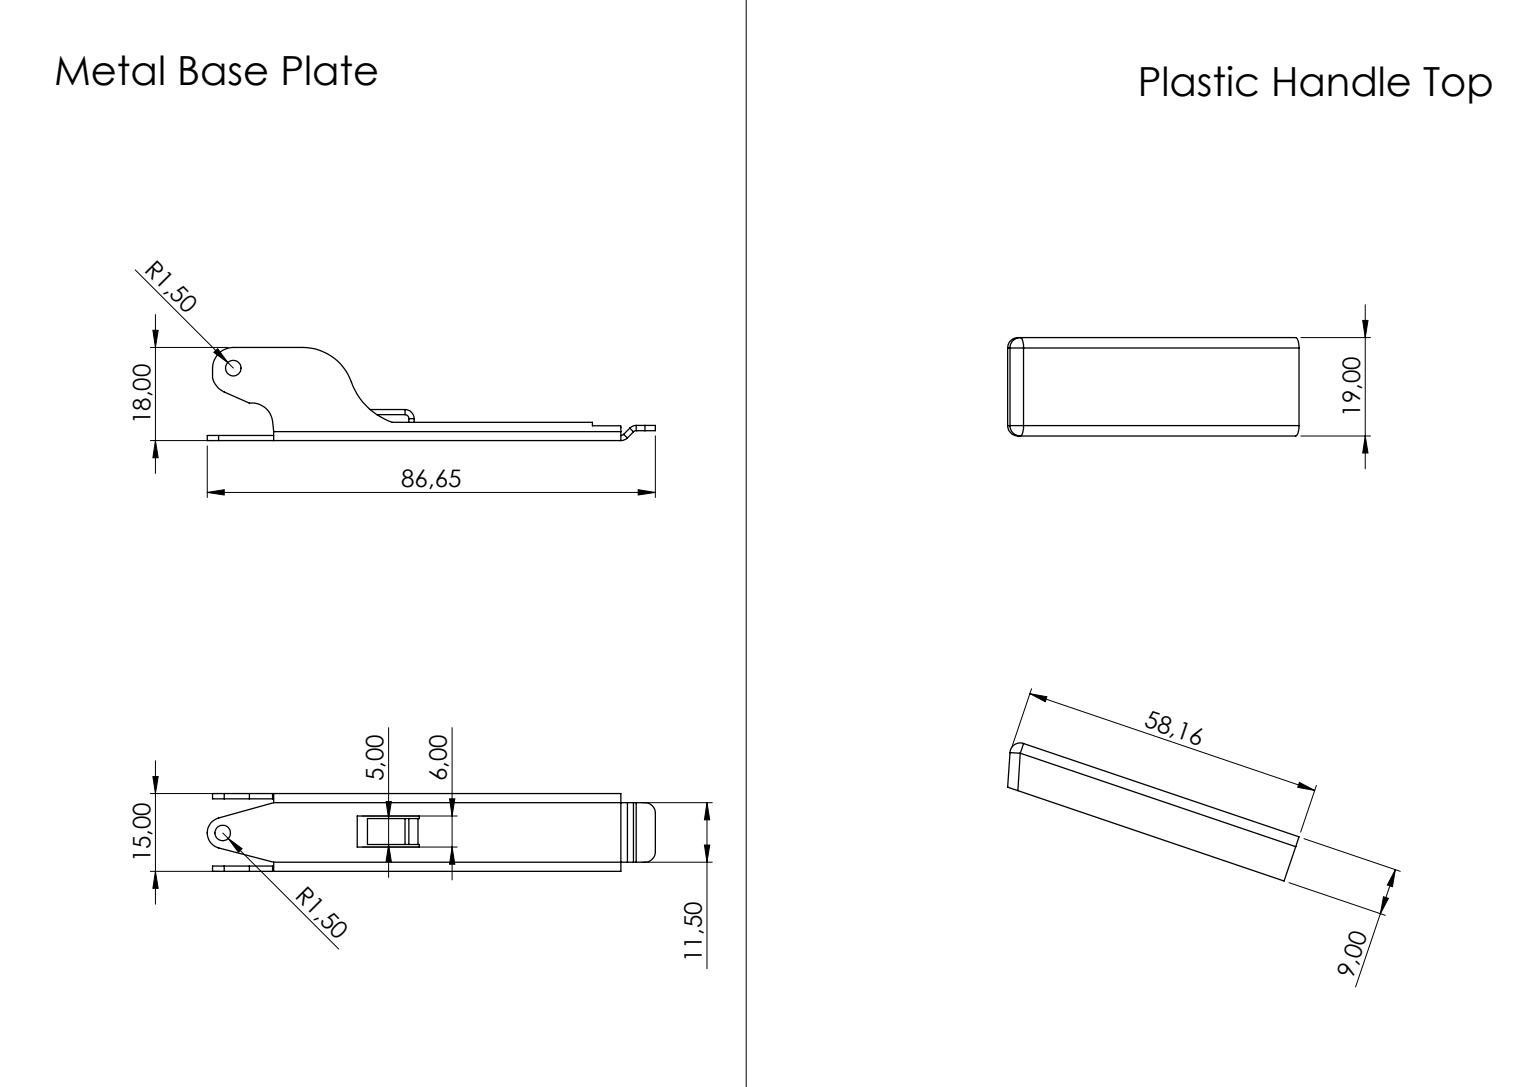
ISO-10303-21;
HEADER;
FILE_DESCRIPTION (('STEP AP214'),
    '1' );
FILE_NAME ('Metal Base Plate.step',
    '2026-10-06T10:23:46',
    ( '' ),
    ( '' ),
    'SwSTEP 2.0',
    'SolidWorks 2020',
    '' );
FILE_SCHEMA (( 'AUTOMOTIVE_DESIGN' ));
ENDSEC;

DATA;
#1=CARTESIAN_POINT ( 'NONE',  ( 35.64099152588522657, -0.6071811381869983704, 82.55501292736997243 ) ) ;
#4=CARTESIAN_POINT ( 'NONE',  ( 32.56606138205700773, 43.35512946304240245, 83.12823623207320622 ) ) ;
#16=EDGE_CURVE ( 'NONE', #3263, #15554, #24734, .T. ) ;
#19=CARTESIAN_POINT ( 'NONE',  ( 35.14099152588522657, 1.392818861812999964, 83.30501292736997243 ) ) ;
#24=ORIENTED_EDGE ( 'NONE', *, *, #17686, .T. ) ;
#31=LINE ( 'NONE', #9973, #22803 ) ;
#41=ORIENTED_EDGE ( 'NONE', *, *, #9883, .F. ) ;
#55=LINE ( 'NONE', #13982, #12355 ) ;
#76=ORIENTED_EDGE ( 'NONE', *, *, #14029, .F. ) ;
#80=CARTESIAN_POINT ( 'NONE',  ( 44.81606138205700063, -25.52563857111379875, 92.39878177866870601 ) ) ;
#89=EDGE_LOOP ( 'NONE', ( #3243, #17530, #4061, #10924 ) ) ;
#101=CARTESIAN_POINT ( 'NONE',  ( 35.64099152588522657, 40.83281886181300280, 79.30501292736983032 ) ) ;
#110=LINE ( 'NONE', #17914, #18667 ) ;
#119=ORIENTED_EDGE ( 'NONE', *, *, #11030, .T. ) ;
#120=VERTEX_POINT ( 'NONE', #3105 ) ;
#128=EDGE_CURVE ( 'NONE', #1147, #21871, #2352, .T. ) ;
#131=VERTEX_POINT ( 'NONE', #14581 ) ;
#133=CARTESIAN_POINT ( 'NONE',  ( 40.64099152588522657, -1.357181138186998925, 80.05501292737000085 ) ) ;
#136=FACE_OUTER_BOUND ( 'NONE', #6898, .T. ) ;
#152=LINE ( 'NONE', #3900, #22918 ) ;
#161=ORIENTED_EDGE ( 'NONE', *, *, #12871, .T. ) ;
#173=DIRECTION ( 'NONE',  ( 0.000000000000000000, 1.000000000000000000, -3.469446951953701358E-15 ) ) ;
#178=LINE ( 'NONE', #16145, #1575 ) ;
#194=VERTEX_POINT ( 'NONE', #1 ) ;
#202=CARTESIAN_POINT ( 'NONE',  ( 44.81606138205700063, 40.34464305740947765, 81.44836866983821722 ) ) ;
#204=ORIENTED_EDGE ( 'NONE', *, *, #17940, .F. ) ;
#217=CARTESIAN_POINT ( 'NONE',  ( 31.81606138205700418, -31.45856502260510013, 77.07494475056050476 ) ) ;
#218=EDGE_LOOP ( 'NONE', ( #9842, #8008, #1464, #22702 ) ) ;
#225=CARTESIAN_POINT ( 'NONE',  ( 30.81606138205700418, -21.15876147765410309, 66.30501292737000085 ) ) ;
#243=EDGE_CURVE ( 'NONE', #17020, #9362, #11367, .T. ) ;
#257=CARTESIAN_POINT ( 'NONE',  ( 34.56606138205700773, 45.04446929126255128, 81.37823623207320622 ) ) ;
#261=EDGE_CURVE ( 'NONE', #11274, #17540, #5561, .T. ) ;
#272=ORIENTED_EDGE ( 'NONE', *, *, #16077, .F. ) ;
#275=DIRECTION ( 'NONE',  ( -1.000000000000000000, -1.734723475976799945E-16, 1.734723475976814737E-16 ) ) ;
#280=CARTESIAN_POINT ( 'NONE',  ( 30.81606138205700418, -0.6071811381869983704, 82.55501292736998664 ) ) ;
#284=EDGE_CURVE ( 'NONE', #21429, #18272, #15214, .T. ) ;
#287=LINE ( 'NONE', #10351, #18422 ) ;
#291=VECTOR ( 'NONE', #3755, 1000.000000000000000 ) ;
#306=ORIENTED_EDGE ( 'NONE', *, *, #2685, .F. ) ;
#330=CIRCLE ( 'NONE', #7350, 1.500000000000001332 ) ;
#332=DIRECTION ( 'NONE',  ( 1.734723475976814737E-16, -1.000000000000000000, 3.491481338843135327E-15 ) ) ;
#334=DIRECTION ( 'NONE',  ( -1.000000000000000000, 0.000000000000000000, 0.000000000000000000 ) ) ;
#337=CARTESIAN_POINT ( 'NONE',  ( 32.56606138205700773, 40.39281886181299797, 83.30501292736984453 ) ) ;
#338=ORIENTED_EDGE ( 'NONE', *, *, #17984, .T. ) ;
#360=EDGE_LOOP ( 'NONE', ( #9313, #7335, #23676, #19391, #21590, #5300, #7158, #3362 ) ) ;
#372=ORIENTED_EDGE ( 'NONE', *, *, #24453, .T. ) ;
#394=ADVANCED_FACE ( 'NONE', ( #12384 ), #4140, .F. ) ;
#395=CARTESIAN_POINT ( 'NONE',  ( 30.81606138205700418, -26.74044063519535186, 82.50501292737007475 ) ) ;
#401=CARTESIAN_POINT ( 'NONE',  ( 38.44255644662678861, -39.60718113818700203, 83.30501292737011454 ) ) ;
#408=DIRECTION ( 'NONE',  ( 0.000000000000000000, 1.000000000000000000, -4.625929269271481378E-15 ) ) ;
#414=FACE_OUTER_BOUND ( 'NONE', #16051, .T. ) ;
#426=AXIS2_PLACEMENT_3D ( 'NONE', #23503, #3937, #7679 ) ;
#437=DIRECTION ( 'NONE',  ( 0.000000000000000000, 1.000000000000000000, -6.938893903907222067E-15 ) ) ;
#441=ORIENTED_EDGE ( 'NONE', *, *, #10566, .F. ) ;
#458=EDGE_CURVE ( 'NONE', #22083, #20938, #22536, .T. ) ;
#464=DIRECTION ( 'NONE',  ( -1.734723475976814737E-16, -3.009265538105065873E-32, -1.000000000000000000 ) ) ;
#491=EDGE_CURVE ( 'NONE', #22735, #4487, #20477, .T. ) ;
#493=ORIENTED_EDGE ( 'NONE', *, *, #7515, .F. ) ;
#503=DIRECTION ( 'NONE',  ( 0.000000000000000000, -3.491481338843135327E-15, -1.000000000000000000 ) ) ;
#507=DIRECTION ( 'NONE',  ( -0.000000000000000000, 1.000000000000000000, 0.000000000000000000 ) ) ;
#508=DIRECTION ( 'NONE',  ( 0.000000000000000000, -3.269436733918100469E-15, -1.000000000000000000 ) ) ;
#511=DIRECTION ( 'NONE',  ( 1.734723475976804876E-16, 3.491481338843135327E-15, 1.000000000000000000 ) ) ;
#516=AXIS2_PLACEMENT_3D ( 'NONE', #2871, #20924, #11140 ) ;
#528=ORIENTED_EDGE ( 'NONE', *, *, #18616, .T. ) ;
#547=DIRECTION ( 'NONE',  ( 0.000000000000000000, -3.491481338843135327E-15, -1.000000000000000000 ) ) ;
#548=DIRECTION ( 'NONE',  ( -8.381647117973248681E-31, -0.7071067811865460184, -0.7071067811865489050 ) ) ;
#571=CYLINDRICAL_SURFACE ( 'NONE', #12870, 1.749999999999998668 ) ;
#574=EDGE_CURVE ( 'NONE', #16761, #23326, #24565, .T. ) ;
#581=CIRCLE ( 'NONE', #14988, 1.500000000000001332 ) ;
#584=EDGE_CURVE ( 'NONE', #10773, #7324, #23762, .T. ) ;
#585=ORIENTED_EDGE ( 'NONE', *, *, #15854, .T. ) ;
#600=AXIS2_PLACEMENT_3D ( 'NONE', #19096, #2975, #3368 ) ;
#636=DIRECTION ( 'NONE',  ( -7.966588320977881105E-33, 1.000000000000000000, -6.123233995736769734E-17 ) ) ;
#643=VERTEX_POINT ( 'NONE', #12347 ) ;
#648=PLANE ( 'NONE',  #1506 ) ;
#654=ORIENTED_EDGE ( 'NONE', *, *, #13211, .F. ) ;
#660=DIRECTION ( 'NONE',  ( -1.000000000000000000, 0.000000000000000000, 1.734723475976804876E-16 ) ) ;
#661=DIRECTION ( 'NONE',  ( -1.000000000000000000, 0.000000000000000000, 1.734723475976804876E-16 ) ) ;
#666=EDGE_CURVE ( 'NONE', #2759, #3821, #18380, .T. ) ;
#668=ORIENTED_EDGE ( 'NONE', *, *, #7604, .F. ) ;
#688=ORIENTED_EDGE ( 'NONE', *, *, #4557, .F. ) ;
#711=EDGE_CURVE ( 'NONE', #7305, #21390, #8216, .T. ) ;
#721=EDGE_CURVE ( 'NONE', #5120, #2117, #13915, .T. ) ;
#724=ORIENTED_EDGE ( 'NONE', *, *, #19582, .F. ) ;
#725=PLANE ( 'NONE',  #8329 ) ;
#729=EDGE_CURVE ( 'NONE', #4335, #24890, #4481, .T. ) ;
#735=VECTOR ( 'NONE', #19670, 1000.000000000000000 ) ;
#752=DIRECTION ( 'NONE',  ( -9.121204216617950752E-31, -0.7071067811865461294, -0.7071067811865490160 ) ) ;
#753=CARTESIAN_POINT ( 'NONE',  ( 30.81606138205700418, -21.15876147765404625, 76.30501292736998664 ) ) ;
#755=ORIENTED_EDGE ( 'NONE', *, *, #12133, .T. ) ;
#789=DIRECTION ( 'NONE',  ( 9.614242282381077875E-31, 0.7071067811865460184, 0.7071067811865489050 ) ) ;
#800=FACE_OUTER_BOUND ( 'NONE', #1702, .T. ) ;
#805=LINE ( 'NONE', #8691, #16582 ) ;
#806=DIRECTION ( 'NONE',  ( -1.000000000000000000, 0.000000000000000000, 2.478176394252580155E-16 ) ) ;
#817=CARTESIAN_POINT ( 'NONE',  ( 43.24475484328152675, -1.357181138186998925, 80.05501292736997243 ) ) ;
#829=ORIENTED_EDGE ( 'NONE', *, *, #19452, .F. ) ;
#830=DIRECTION ( 'NONE',  ( -1.734723475976809806E-16, 0.000000000000000000, -1.000000000000000000 ) ) ;
#835=VECTOR ( 'NONE', #10940, 1000.000000000000000 ) ;
#836=CARTESIAN_POINT ( 'NONE',  ( 31.81606138205700418, -34.55876147765410167, 66.30501292737000085 ) ) ;
#841=ORIENTED_EDGE ( 'NONE', *, *, #2654, .F. ) ;
#846=VECTOR ( 'NONE', #7817, 1000.000000000000000 ) ;
#856=DIRECTION ( 'NONE',  ( 0.000000000000000000, 0.000000000000000000, -1.000000000000000000 ) ) ;
#857=DIRECTION ( 'NONE',  ( -1.734723475976879818E-16, 1.000000000000000000, -4.343580702399009298E-14 ) ) ;
#885=DIRECTION ( 'NONE',  ( 0.000000000000000000, 0.000000000000000000, -1.000000000000000000 ) ) ;
#901=AXIS2_PLACEMENT_3D ( 'NONE', #10296, #24061, #6178 ) ;
#903=FACE_BOUND ( 'NONE', #23651, .T. ) ;
#913=ORIENTED_EDGE ( 'NONE', *, *, #13102, .T. ) ;
#924=VECTOR ( 'NONE', #10529, 1000.000000000000000 ) ;
#928=VECTOR ( 'NONE', #2718, 1000.000000000000000 ) ;
#934=CARTESIAN_POINT ( 'NONE',  ( 30.81606138205700418, 34.87886987267149408, 80.75501292736984738 ) ) ;
#938=AXIS2_PLACEMENT_3D ( 'NONE', #817, #24387, #22469 ) ;
#942=FACE_OUTER_BOUND ( 'NONE', #19532, .T. ) ;
#956=VECTOR ( 'NONE', #7416, 1000.000000000000114 ) ;
#957=CARTESIAN_POINT ( 'NONE',  ( 30.81606138205700418, -1.357181138186998925, 79.30501292737000085 ) ) ;
#959=ORIENTED_EDGE ( 'NONE', *, *, #4050, .T. ) ;
#972=CARTESIAN_POINT ( 'NONE',  ( 35.14099152588522657, -10.60718113818700026, 83.30501292737001506 ) ) ;
#975=DIRECTION ( 'NONE',  ( -1.000000000000000000, 0.000000000000000000, 1.734723475976804876E-16 ) ) ;
#983=CARTESIAN_POINT ( 'NONE',  ( 44.06606138205700063, 40.39281886181299797, 82.55501292736983032 ) ) ;
#989=VECTOR ( 'NONE', #18459, 1000.000000000000000 ) ;
#994=EDGE_CURVE ( 'NONE', #25303, #14052, #9742, .T. ) ;
#996=CARTESIAN_POINT ( 'NONE',  ( 44.81606138205700063, -30.95005513552129983, 81.04249030099066431 ) ) ;
#1021=PLANE ( 'NONE',  #24911 ) ;
#1038=EDGE_LOOP ( 'NONE', ( #11997, #17760, #10721, #8351 ) ) ;
#1045=ORIENTED_EDGE ( 'NONE', *, *, #24087, .F. ) ;
#1060=DIRECTION ( 'NONE',  ( 0.000000000000000000, -9.251858538542962756E-15, -1.000000000000000000 ) ) ;
#1083=ORIENTED_EDGE ( 'NONE', *, *, #18532, .F. ) ;
#1088=FACE_OUTER_BOUND ( 'NONE', #12606, .T. ) ;
#1098=ORIENTED_EDGE ( 'NONE', *, *, #18616, .F. ) ;
#1102=AXIS2_PLACEMENT_3D ( 'NONE', #20396, #12433, #2726 ) ;
#1111=CARTESIAN_POINT ( 'NONE',  ( 44.06606138205700063, 43.35512946304240245, 82.37823623207322044 ) ) ;
#1114=DIRECTION ( 'NONE',  ( 0.000000000000000000, -4.116873784215925398E-15, -1.000000000000000000 ) ) ;
#1115=CARTESIAN_POINT ( 'NONE',  ( 44.81606138205700063, -38.55876147765349771, 84.30501292737325514 ) ) ;
#1140=CARTESIAN_POINT ( 'NONE',  ( 17.31606138205699708, 42.46194149498198556, 81.44836866983821722 ) ) ;
#1143=CARTESIAN_POINT ( 'NONE',  ( 30.81606138205700418, -10.60718113818700026, 84.30501292737000085 ) ) ;
#1147=VERTEX_POINT ( 'NONE', #202 ) ;
#1154=EDGE_LOOP ( 'NONE', ( #13545, #20999, #8153, #9864 ) ) ;
#1162=EDGE_LOOP ( 'NONE', ( #24133, #21843, #12662, #15082 ) ) ;
#1178=PLANE ( 'NONE',  #7609 ) ;
#1201=DIRECTION ( 'NONE',  ( 1.000000000000000000, 1.734723475976804876E-16, -1.734723475976814737E-16 ) ) ;
#1205=VERTEX_POINT ( 'NONE', #14003 ) ;
#1219=EDGE_CURVE ( 'NONE', #1205, #10773, #20042, .T. ) ;
#1228=VECTOR ( 'NONE', #9593, 1000.000000000000000 ) ;
#1251=EDGE_CURVE ( 'NONE', #3863, #5274, #4832, .T. ) ;
#1257=CARTESIAN_POINT ( 'NONE',  ( 32.56606138205700773, 43.35512946304240245, 82.37823623207322044 ) ) ;
#1276=ORIENTED_EDGE ( 'NONE', *, *, #23502, .F. ) ;
#1292=ORIENTED_EDGE ( 'NONE', *, *, #10707, .F. ) ;
#1300=EDGE_CURVE ( 'NONE', #23758, #7648, #9233, .T. ) ;
#1306=DIRECTION ( 'NONE',  ( -1.734723475976804876E-16, -3.469446951953610245E-15, -1.000000000000000000 ) ) ;
#1317=AXIS2_PLACEMENT_3D ( 'NONE', #11954, #4341, #2385 ) ;
#1327=CIRCLE ( 'NONE', #20258, 1.750000000000001554 ) ;
#1329=ORIENTED_EDGE ( 'NONE', *, *, #12339, .T. ) ;
#1335=ORIENTED_EDGE ( 'NONE', *, *, #4372, .F. ) ;
#1338=CARTESIAN_POINT ( 'NONE',  ( 30.81606138205700418, 1.142818861812999742, 84.30501292737000085 ) ) ;
#1346=ORIENTED_EDGE ( 'NONE', *, *, #18533, .T. ) ;
#1353=CARTESIAN_POINT ( 'NONE',  ( 30.81606138205700418, 40.39281886181299797, 82.55501292736983032 ) ) ;
#1356=VECTOR ( 'NONE', #1201, 1000.000000000000000 ) ;
#1360=ORIENTED_EDGE ( 'NONE', *, *, #12429, .F. ) ;
#1370=ORIENTED_EDGE ( 'NONE', *, *, #10698, .F. ) ;
#1388=DIRECTION ( 'NONE',  ( 0.000000000000000000, 1.000000000000000000, -3.469446951953614189E-15 ) ) ;
#1402=LINE ( 'NONE', #7459, #2527 ) ;
#1445=LINE ( 'NONE', #15479, #291 ) ;
#1451=EDGE_CURVE ( 'NONE', #9965, #13296, #11792, .T. ) ;
#1463=ORIENTED_EDGE ( 'NONE', *, *, #7053, .F. ) ;
#1464=ORIENTED_EDGE ( 'NONE', *, *, #574, .T. ) ;
#1482=ORIENTED_EDGE ( 'NONE', *, *, #15615, .T. ) ;
#1487=DIRECTION ( 'NONE',  ( 0.000000000000000000, 1.000000000000000000, -2.775557561562891351E-15 ) ) ;
#1502=DIRECTION ( 'NONE',  ( -1.000000000000000000, 0.000000000000000000, 0.000000000000000000 ) ) ;
#1506=AXIS2_PLACEMENT_3D ( 'NONE', #4542, #12406, #10968 ) ;
#1539=AXIS2_PLACEMENT_3D ( 'NONE', #8047, #8296, #12174 ) ;
#1548=FACE_OUTER_BOUND ( 'NONE', #2716, .T. ) ;
#1552=CARTESIAN_POINT ( 'NONE',  ( 41.14099152588522657, -10.60718113818700026, 84.30501292737000085 ) ) ;
#1560=CARTESIAN_POINT ( 'NONE',  ( 32.56606138205700773, 40.70347903359284913, 83.30501292736984453 ) ) ;
#1563=PLANE ( 'NONE',  #17422 ) ;
#1565=DIRECTION ( 'NONE',  ( 0.2672894156317878744, -0.9636162972320556630, 3.318080997173179155E-15 ) ) ;
#1575=VECTOR ( 'NONE', #11801, 1000.000000000000000 ) ;
#1577=VERTEX_POINT ( 'NONE', #1586 ) ;
#1586=CARTESIAN_POINT ( 'NONE',  ( 45.81606138205700063, 40.39281886181299797, 81.75501292736983316 ) ) ;
#1591=CARTESIAN_POINT ( 'NONE',  ( 44.81606138205700063, -26.74044063519535186, 84.30501292737007191 ) ) ;
#1596=EDGE_LOOP ( 'NONE', ( #4066, #21811, #10775, #18023 ) ) ;
#1598=EDGE_CURVE ( 'NONE', #15541, #120, #287, .T. ) ;
#1622=DIRECTION ( 'NONE',  ( 1.000000000000000000, 2.065146995210479765E-16, -1.734723475976814737E-16 ) ) ;
#1627=EDGE_CURVE ( 'NONE', #9965, #22735, #22195, .T. ) ;
#1650=EDGE_CURVE ( 'NONE', #12300, #7324, #14225, .T. ) ;
#1668=DIRECTION ( 'NONE',  ( -1.734723475976804876E-16, -3.491481338843135327E-15, -1.000000000000000000 ) ) ;
#1674=EDGE_CURVE ( 'NONE', #5806, #9258, #2099, .T. ) ;
#1675=ADVANCED_FACE ( 'NONE', ( #414 ), #8427, .F. ) ;
#1686=EDGE_CURVE ( 'NONE', #4506, #22728, #20142, .T. ) ;
#1702=EDGE_LOOP ( 'NONE', ( #16971, #18877, #24015, #20126 ) ) ;
#1715=FACE_OUTER_BOUND ( 'NONE', #18455, .T. ) ;
#1721=DIRECTION ( 'NONE',  ( 1.000000000000000000, 0.000000000000000000, 0.000000000000000000 ) ) ;
#1726=DIRECTION ( 'NONE',  ( 0.000000000000000000, 1.000000000000000000, -4.625929269271481378E-15 ) ) ;
#1743=VECTOR ( 'NONE', #5542, 1000.000000000000000 ) ;
#1747=DIRECTION ( 'NONE',  ( 0.000000000000000000, 0.000000000000000000, 1.000000000000000000 ) ) ;
#1759=ORIENTED_EDGE ( 'NONE', *, *, #12427, .T. ) ;
#1760=AXIS2_PLACEMENT_3D ( 'NONE', #16947, #3023, #830 ) ;
#1766=MECHANICAL_DESIGN_GEOMETRIC_PRESENTATION_REPRESENTATION('',(#17014),#3838);
#1815=ORIENTED_EDGE ( 'NONE', *, *, #14904, .T. ) ;
#1838=CARTESIAN_POINT ( 'NONE',  ( 31.81606138205700418, -11.72563467517899838, 72.98595903681224684 ) ) ;
#1849=DIRECTION ( 'NONE',  ( -1.734723475976804876E-16, -3.469446951953610245E-15, -1.000000000000000000 ) ) ;
#1854=CARTESIAN_POINT ( 'NONE',  ( 38.41621794735363693, -36.60729675983900222, 83.30501292737011454 ) ) ;
#1862=EDGE_LOOP ( 'NONE', ( #9658, #372, #668, #7998 ) ) ;
#1884=DIRECTION ( 'NONE',  ( 0.000000000000000000, -1.000000000000000000, 3.491481338843135327E-15 ) ) ;
#1908=DIRECTION ( 'NONE',  ( 1.000000000000000000, 1.734723475976804876E-16, -1.734723475976814737E-16 ) ) ;
#1910=AXIS2_PLACEMENT_3D ( 'NONE', #19470, #15097, #25253 ) ;
#1917=CARTESIAN_POINT ( 'NONE',  ( 44.06606138205700063, -26.74044063519535186, 82.55501292737007191 ) ) ;
#1924=EDGE_LOOP ( 'NONE', ( #4738, #10941, #16863, #9235 ) ) ;
#1928=CIRCLE ( 'NONE', #23314, 3.999999999999899636 ) ;
#1948=EDGE_CURVE ( 'NONE', #8461, #10371, #20520, .T. ) ;
#1961=CARTESIAN_POINT ( 'NONE',  ( 31.81606138205700418, 34.87886987267149408, 66.30501292737000085 ) ) ;
#1971=VERTEX_POINT ( 'NONE', #3751 ) ;
#1972=PLANE ( 'NONE',  #2191 ) ;
#1989=CIRCLE ( 'NONE', #5293, 3.999999999999899636 ) ;
#2000=AXIS2_PLACEMENT_3D ( 'NONE', #9286, #12766, #22537 ) ;
#2008=EDGE_CURVE ( 'NONE', #15541, #11322, #5825, .T. ) ;
#2018=DIRECTION ( 'NONE',  ( 1.000000000000000000, 1.734723475976805122E-16, -1.734723475976814737E-16 ) ) ;
#2019=ADVANCED_FACE ( 'NONE', ( #11764 ), #19345, .F. ) ;
#2020=ADVANCED_FACE ( 'NONE', ( #19218 ), #21279, .F. ) ;
#2028=VECTOR ( 'NONE', #18443, 1000.000000000000000 ) ;
#2029=ORIENTED_EDGE ( 'NONE', *, *, #24650, .F. ) ;
#2041=AXIS2_PLACEMENT_3D ( 'NONE', #23198, #13678, #15348 ) ;
#2045=CARTESIAN_POINT ( 'NONE',  ( 45.81606138205700063, -21.15876147765404625, 76.30501292736998664 ) ) ;
#2054=EDGE_CURVE ( 'NONE', #16440, #19362, #7708, .T. ) ;
#2063=PLANE ( 'NONE',  #8048 ) ;
#2066=DIRECTION ( 'NONE',  ( -1.000000000000000000, 0.000000000000000000, 0.000000000000000000 ) ) ;
#2099=LINE ( 'NONE', #23861, #23765 ) ;
#2103=CARTESIAN_POINT ( 'NONE',  ( 44.81606138205700063, -34.67340937580780036, 71.26505871168839690 ) ) ;
#2117=VERTEX_POINT ( 'NONE', #3376 ) ;
#2140=DIRECTION ( 'NONE',  ( -1.000000000000000000, 6.018531076210130433E-31, 1.734723475976804876E-16 ) ) ;
#2143=LINE ( 'NONE', #6156, #6973 ) ;
#2162=CARTESIAN_POINT ( 'NONE',  ( 44.81606138205700063, -11.72563467517899838, 72.98595903681223263 ) ) ;
#2191=AXIS2_PLACEMENT_3D ( 'NONE', #5859, #11796, #547 ) ;
#2202=CARTESIAN_POINT ( 'NONE',  ( 44.81606138205700063, 40.39281886181299797, 81.44836866983821722 ) ) ;
#2204=AXIS2_PLACEMENT_3D ( 'NONE', #3710, #15442, #24951 ) ;
#2219=CIRCLE ( 'NONE', #23197, 1.500000000000001332 ) ;
#2230=CARTESIAN_POINT ( 'NONE',  ( 44.81606138205700063, -31.45856502260510013, 77.07494475056050476 ) ) ;
#2233=EDGE_CURVE ( 'NONE', #24557, #120, #7668, .T. ) ;
#2238=VECTOR ( 'NONE', #2346, 1000.000000000000000 ) ;
#2240=ORIENTED_EDGE ( 'NONE', *, *, #6083, .T. ) ;
#2245=VERTEX_POINT ( 'NONE', #19762 ) ;
#2246=EDGE_CURVE ( 'NONE', #4432, #8461, #1928, .T. ) ;
#2254=VERTEX_POINT ( 'NONE', #19254 ) ;
#2256=DIRECTION ( 'NONE',  ( 1.000000000000000000, 2.168404344971010101E-16, -1.734723475976814737E-16 ) ) ;
#2269=DIRECTION ( 'NONE',  ( 0.000000000000000000, 1.000000000000000000, -3.304235192336775512E-15 ) ) ;
#2282=DIRECTION ( 'NONE',  ( 1.734723475976804876E-16, 3.491481338843135327E-15, 1.000000000000000000 ) ) ;
#2290=VERTEX_POINT ( 'NONE', #11411 ) ;
#2291=DIRECTION ( 'NONE',  ( -1.734723475976804876E-16, -3.552713678800500140E-15, -1.000000000000000000 ) ) ;
#2292=ADVANCED_FACE ( 'NONE', ( #1715 ), #3926, .F. ) ;
#2314=LINE ( 'NONE', #8131, #13998 ) ;
#2321=EDGE_CURVE ( 'NONE', #13207, #3634, #2356, .T. ) ;
#2330=ADVANCED_FACE ( 'NONE', ( #18466 ), #12564, .T. ) ;
#2334=AXIS2_PLACEMENT_3D ( 'NONE', #7760, #17297, #7500 ) ;
#2340=DIRECTION ( 'NONE',  ( 1.734723475976804876E-16, 3.491481338843135327E-15, 1.000000000000000000 ) ) ;
#2346=DIRECTION ( 'NONE',  ( -0.000000000000000000, -0.000000000000000000, -1.000000000000000000 ) ) ;
#2347=DIRECTION ( 'NONE',  ( 1.734723475976804876E-16, 3.469446951953610245E-15, 1.000000000000000000 ) ) ;
#2352=CIRCLE ( 'NONE', #12251, 1.000000000000000888 ) ;
#2354=CIRCLE ( 'NONE', #14697, 12.59999999999999964 ) ;
#2356=LINE ( 'NONE', #4314, #3984 ) ;
#2385=DIRECTION ( 'NONE',  ( 0.000000000000000000, 0.000000000000000000, 1.000000000000000000 ) ) ;
#2390=CARTESIAN_POINT ( 'NONE',  ( 30.81606138205700418, 40.34464305740947054, 81.44836866983821722 ) ) ;
#2396=DIRECTION ( 'NONE',  ( 0.000000000000000000, 1.000000000000000000, 0.000000000000000000 ) ) ;
#2422=CARTESIAN_POINT ( 'NONE',  ( 30.81606138205700418, -38.55876147765410167, 70.30501292737011454 ) ) ;
#2442=PLANE ( 'NONE',  #3297 ) ;
#2446=CARTESIAN_POINT ( 'NONE',  ( 35.52536905565747105, -37.40916500673439771, 83.30501292737011454 ) ) ;
#2463=CARTESIAN_POINT ( 'NONE',  ( 31.81606138205700418, -21.15876147765404625, 76.30501292736998664 ) ) ;
#2467=EDGE_CURVE ( 'NONE', #14211, #17608, #8557, .T. ) ;
#2473=DIRECTION ( 'NONE',  ( -1.000000000000000000, -2.168404344971060144E-16, 1.734723475976814737E-16 ) ) ;
#2479=CARTESIAN_POINT ( 'NONE',  ( 31.81606138205700418, -21.15876147765410309, 66.30501292737000085 ) ) ;
#2481=ORIENTED_EDGE ( 'NONE', *, *, #12234, .F. ) ;
#2495=ORIENTED_EDGE ( 'NONE', *, *, #14029, .T. ) ;
#2496=VERTEX_POINT ( 'NONE', #24614 ) ;
#2499=UNCERTAINTY_MEASURE_WITH_UNIT (LENGTH_MEASURE( 1.000000000000000082E-05 ), #2755, 'distance_accuracy_value', 'NONE');
#2502=ORIENTED_EDGE ( 'NONE', *, *, #12738, .T. ) ;
#2506=ORIENTED_EDGE ( 'NONE', *, *, #7660, .T. ) ;
#2521=EDGE_CURVE ( 'NONE', #3225, #11274, #11125, .T. ) ;
#2522=CARTESIAN_POINT ( 'NONE',  ( 45.81606138205700063, -31.45856502260500065, 77.07494475056050476 ) ) ;
#2527=VECTOR ( 'NONE', #7330, 1000.000000000000000 ) ;
#2531=VERTEX_POINT ( 'NONE', #5197 ) ;
#2548=FACE_OUTER_BOUND ( 'NONE', #14715, .T. ) ;
#2551=VERTEX_POINT ( 'NONE', #6996 ) ;
#2555=ORIENTED_EDGE ( 'NONE', *, *, #9425, .T. ) ;
#2556=ORIENTED_EDGE ( 'NONE', *, *, #24059, .F. ) ;
#2565=CARTESIAN_POINT ( 'NONE',  ( 44.06606138205700063, 43.35512946304240245, 82.37823623207322044 ) ) ;
#2575=DIRECTION ( 'NONE',  ( -1.000000000000000000, -1.734723475976804876E-16, 1.734723475976814737E-16 ) ) ;
#2581=AXIS2_PLACEMENT_3D ( 'NONE', #8423, #2473, #21813 ) ;
#2602=DIRECTION ( 'NONE',  ( 0.000000000000000000, -1.000000000000000000, 3.469446951953701358E-15 ) ) ;
#2603=AXIS2_PLACEMENT_3D ( 'NONE', #7492, #5819, #11370 ) ;
#2605=ADVANCED_FACE ( 'NONE', ( #2988 ), #7254, .T. ) ;
#2607=CARTESIAN_POINT ( 'NONE',  ( 31.81606138205700418, -26.74044063519535186, 82.55501292737007191 ) ) ;
#2617=VECTOR ( 'NONE', #17651, 1000.000000000000000 ) ;
#2644=FACE_OUTER_BOUND ( 'NONE', #7408, .T. ) ;
#2648=CARTESIAN_POINT ( 'NONE',  ( 35.64099152588522657, 0.3928188618129990761, 73.02501292736999972 ) ) ;
#2654=EDGE_CURVE ( 'NONE', #23852, #1577, #8534, .T. ) ;
#2674=CARTESIAN_POINT ( 'NONE',  ( 40.64099152588522657, 1.392818861812999964, 83.30501292736997243 ) ) ;
#2683=PLANE ( 'NONE',  #14439 ) ;
#2685=EDGE_CURVE ( 'NONE', #21676, #24723, #1445, .T. ) ;
#2716=EDGE_LOOP ( 'NONE', ( #23000, #13285, #5049, #13767 ) ) ;
#2718=DIRECTION ( 'NONE',  ( -1.000000000000000000, -1.734723475976804876E-16, 1.734723475976814737E-16 ) ) ;
#2726=DIRECTION ( 'NONE',  ( -1.734723475976804876E-16, 1.000000000000000000, 0.000000000000000000 ) ) ;
#2732=VECTOR ( 'NONE', #21409, 1000.000000000000114 ) ;
#2750=FACE_OUTER_BOUND ( 'NONE', #24828, .T. ) ;
#2755=( LENGTH_UNIT ( ) NAMED_UNIT ( * ) SI_UNIT ( .MILLI., .METRE. ) );
#2759=VERTEX_POINT ( 'NONE', #19219 ) ;
#2760=FACE_OUTER_BOUND ( 'NONE', #11147, .T. ) ;
#2765=DIRECTION ( 'NONE',  ( 1.734723475976804876E-16, 3.252606517456515274E-15, 1.000000000000000000 ) ) ;
#2777=EDGE_CURVE ( 'NONE', #24921, #120, #12252, .T. ) ;
#2787=EDGE_CURVE ( 'NONE', #11322, #11291, #11378, .T. ) ;
#2791=LINE ( 'NONE', #7191, #18097 ) ;
#2793=VECTOR ( 'NONE', #4600, 1000.000000000000000 ) ;
#2799=LINE ( 'NONE', #2674, #18908 ) ;
#2814=CARTESIAN_POINT ( 'NONE',  ( 41.14099152588522657, 1.392818861812999964, 83.30501292736997243 ) ) ;
#2839=DIRECTION ( 'NONE',  ( -1.000000000000000000, -1.734723475976814737E-16, 6.878321229954450795E-31 ) ) ;
#2842=DIRECTION ( 'NONE',  ( 0.2503287245161955887, 0.9681609007195522976, -3.423740829372836395E-15 ) ) ;
#2845=CARTESIAN_POINT ( 'NONE',  ( 38.41621794735363693, -36.60729675983900222, 83.30501292737011454 ) ) ;
#2851=DIRECTION ( 'NONE',  ( 0.2672894156317878744, -0.9636162972320556630, 3.318080997173179155E-15 ) ) ;
#2855=DIRECTION ( 'NONE',  ( 1.000000000000000000, 1.734723475976804876E-16, -1.734723475976814737E-16 ) ) ;
#2861=LINE ( 'NONE', #5074, #22572 ) ;
#2870=FACE_BOUND ( 'NONE', #22230, .T. ) ;
#2871=CARTESIAN_POINT ( 'NONE',  ( 41.14099152588523367, -10.60718113818700026, 93.30501292736998664 ) ) ;
#2872=VECTOR ( 'NONE', #15685, 1000.000000000000000 ) ;
#2883=DIRECTION ( 'NONE',  ( 0.000000000000000000, 1.000000000000000000, 7.930164461608253340E-15 ) ) ;
#2889=VECTOR ( 'NONE', #10378, 1000.000000000000000 ) ;
#2896=DIRECTION ( 'NONE',  ( -1.000000000000000000, -2.168404344971010101E-16, 1.734723475976814737E-16 ) ) ;
#2921=EDGE_CURVE ( 'NONE', #16440, #13002, #12398, .T. ) ;
#2926=LINE ( 'NONE', #18534, #16420 ) ;
#2931=DIRECTION ( 'NONE',  ( 1.000000000000000000, 0.000000000000000000, 0.000000000000000000 ) ) ;
#2939=CARTESIAN_POINT ( 'NONE',  ( 31.81606138205700418, -38.55876147765410167, 72.21586839016146087 ) ) ;
#2947=AXIS2_PLACEMENT_3D ( 'NONE', #6664, #18149, #4614 ) ;
#2948=CARTESIAN_POINT ( 'NONE',  ( 45.81606138205700063, -34.55876147765410167, 66.30501292737000085 ) ) ;
#2960=CARTESIAN_POINT ( 'NONE',  ( 35.64099152588522657, -1.357181138186998925, 80.05501292737000085 ) ) ;
#2973=EDGE_LOOP ( 'NONE', ( #14866, #6361, #19579, #5404 ) ) ;
#2975=DIRECTION ( 'NONE',  ( -1.000000000000000000, -1.734723475976804876E-16, 1.734723475976814737E-16 ) ) ;
#2978=VECTOR ( 'NONE', #19951, 1000.000000000000000 ) ;
#2981=CARTESIAN_POINT ( 'NONE',  ( 44.06606138205700063, 43.35512946304240245, 83.12823623207320622 ) ) ;
#2982=EDGE_CURVE ( 'NONE', #7462, #1147, #19860, .T. ) ;
#2987=PLANE ( 'NONE',  #16591 ) ;
#2988=FACE_OUTER_BOUND ( 'NONE', #3836, .T. ) ;
#3007=ORIENTED_EDGE ( 'NONE', *, *, #25106, .F. ) ;
#3014=EDGE_CURVE ( 'NONE', #4268, #13492, #16450, .T. ) ;
#3023=DIRECTION ( 'NONE',  ( 1.000000000000000000, 4.336808689942014655E-17, -1.734723475976809806E-16 ) ) ;
#3032=LINE ( 'NONE', #16384, #19445 ) ;
#3038=LINE ( 'NONE', #16962, #4625 ) ;
#3062=DIRECTION ( 'NONE',  ( -1.734723475976804876E-16, -3.269436733918100469E-15, -1.000000000000000000 ) ) ;
#3067=AXIS2_PLACEMENT_3D ( 'NONE', #2981, #12801, #8814 ) ;
#3076=EDGE_LOOP ( 'NONE', ( #12755, #11807, #21212, #5375 ) ) ;
#3082=VECTOR ( 'NONE', #636, 1000.000000000000000 ) ;
#3086=CARTESIAN_POINT ( 'NONE',  ( 35.64099152588522657, 1.142818861812999742, 82.55501292736997243 ) ) ;
#3096=LINE ( 'NONE', #16249, #7363 ) ;
#3105=CARTESIAN_POINT ( 'NONE',  ( 32.56606138205700773, 41.63025572888945192, 83.79244979444629848 ) ) ;
#3117=DIRECTION ( 'NONE',  ( -1.734723475976804876E-16, 1.000000000000000000, 0.000000000000000000 ) ) ;
#3121=DIRECTION ( 'NONE',  ( -1.734723475976804876E-16, 1.000000000000000000, 0.000000000000000000 ) ) ;
#3126=CARTESIAN_POINT ( 'NONE',  ( 30.81606138205700418, -8.607181138186998481, 79.30501292737000085 ) ) ;
#3154=DIRECTION ( 'NONE',  ( 0.000000000000000000, -1.000000000000000000, 0.000000000000000000 ) ) ;
#3157=DIRECTION ( 'NONE',  ( -1.734723475976814737E-16, 1.000000000000000000, -3.491481338843135327E-15 ) ) ;
#3162=PRODUCT_DEFINITION ( 'UNKNOWN', '', #17057, #4104 ) ;
#3163=DIRECTION ( 'NONE',  ( -1.734723475976804876E-16, -3.491481338843135327E-15, -1.000000000000000000 ) ) ;
#3165=CIRCLE ( 'NONE', #16325, 1.750000000000001554 ) ;
#3171=VECTOR ( 'NONE', #12539, 1000.000000000000000 ) ;
#3173=ORIENTED_EDGE ( 'NONE', *, *, #11868, .F. ) ;
#3178=DIRECTION ( 'NONE',  ( 1.000000000000000000, 1.734723475976805122E-16, -1.734723475976814737E-16 ) ) ;
#3182=DIRECTION ( 'NONE',  ( 0.9636162972320556630, 0.2672894156317878744, -1.100396788012901859E-15 ) ) ;
#3183=DIRECTION ( 'NONE',  ( 8.791731484610113542E-17, -0.9135454576426023099, -0.4067366430757970996 ) ) ;
#3184=CARTESIAN_POINT ( 'NONE',  ( 40.64099152588523367, -1.357181138186998925, 88.30501292736998664 ) ) ;
#3186=VECTOR ( 'NONE', #14654, 1000.000000000000000 ) ;
#3189=DIRECTION ( 'NONE',  ( -1.734723475976804876E-16, -3.491481338843135327E-15, -1.000000000000000000 ) ) ;
#3191=EDGE_LOOP ( 'NONE', ( #14794, #22561, #441, #24466 ) ) ;
#3195=ORIENTED_EDGE ( 'NONE', *, *, #16006, .F. ) ;
#3201=VECTOR ( 'NONE', #4598, 1000.000000000000000 ) ;
#3225=VERTEX_POINT ( 'NONE', #25223 ) ;
#3240=DIRECTION ( 'NONE',  ( -1.000000000000000000, -1.734723475976804876E-16, 1.734723475976814737E-16 ) ) ;
#3243=ORIENTED_EDGE ( 'NONE', *, *, #15936, .F. ) ;
#3263=VERTEX_POINT ( 'NONE', #3475 ) ;
#3267=VECTOR ( 'NONE', #15116, 1000.000000000000000 ) ;
#3273=EDGE_CURVE ( 'NONE', #10220, #16812, #5284, .T. ) ;
#3281=ORIENTED_EDGE ( 'NONE', *, *, #994, .F. ) ;
#3282=CARTESIAN_POINT ( 'NONE',  ( 45.81606138205700063, -34.55876147765410167, 70.30501292737000085 ) ) ;
#3288=ORIENTED_EDGE ( 'NONE', *, *, #22449, .T. ) ;
#3289=VECTOR ( 'NONE', #2340, 1000.000000000000000 ) ;
#3297=AXIS2_PLACEMENT_3D ( 'NONE', #10319, #507, #8394 ) ;
#3321=DIRECTION ( 'NONE',  ( -2.290324355028189071E-16, 0.4067366430757970996, -0.9135454576426023099 ) ) ;
#3323=ORIENTED_EDGE ( 'NONE', *, *, #1674, .T. ) ;
#3343=FACE_OUTER_BOUND ( 'NONE', #3702, .T. ) ;
#3348=DIRECTION ( 'NONE',  ( 1.734723475976804876E-16, 3.469446951953610245E-15, 1.000000000000000000 ) ) ;
#3351=EDGE_LOOP ( 'NONE', ( #7734, #12715, #5817, #24669 ) ) ;
#3362=ORIENTED_EDGE ( 'NONE', *, *, #7097, .F. ) ;
#3368=DIRECTION ( 'NONE',  ( -1.734723475976804876E-16, 1.000000000000000000, 0.000000000000000000 ) ) ;
#3376=CARTESIAN_POINT ( 'NONE',  ( 31.81606138205700418, 40.34464305740947054, 81.44836866983821722 ) ) ;
#3383=LINE ( 'NONE', #20914, #20316 ) ;
#3395=VERTEX_POINT ( 'NONE', #20080 ) ;
#3406=AXIS2_PLACEMENT_3D ( 'NONE', #19803, #2765, #3154 ) ;
#3408=CARTESIAN_POINT ( 'NONE',  ( 30.81606138205700773, 34.87886987267149408, 81.44836866983821722 ) ) ;
#3414=LINE ( 'NONE', #13088, #956 ) ;
#3423=AXIS2_PLACEMENT_3D ( 'NONE', #16922, #12809, #1060 ) ;
#3430=ORIENTED_EDGE ( 'NONE', *, *, #6322, .F. ) ;
#3443=LINE ( 'NONE', #9262, #8327 ) ;
#3465=FILL_AREA_STYLE ('',( #17378 ) ) ;
#3472=DIRECTION ( 'NONE',  ( 1.734723475976804876E-16, 3.491481338843135327E-15, 1.000000000000000000 ) ) ;
#3475=CARTESIAN_POINT ( 'NONE',  ( 41.32070064951228971, -37.35828293338759920, 83.30501292737011454 ) ) ;
#3501=DIRECTION ( 'NONE',  ( -1.000000000000000000, -1.734723475976804876E-16, 1.734723475976814737E-16 ) ) ;
#3511=LINE ( 'NONE', #11385, #10243 ) ;
#3518=DIRECTION ( 'NONE',  ( 1.734723475976804876E-16, 3.491481338843135327E-15, 1.000000000000000000 ) ) ;
#3529=EDGE_CURVE ( 'NONE', #14213, #21871, #21890, .T. ) ;
#3545=PLANE ( 'NONE',  #426 ) ;
#3553=CARTESIAN_POINT ( 'NONE',  ( 31.81606138205700418, 24.50429740018177682, 101.9912164131601457 ) ) ;
#3560=CARTESIAN_POINT ( 'NONE',  ( 45.81606138205700063, -33.05876147765410167, 70.30501292737000085 ) ) ;
#3582=CARTESIAN_POINT ( 'NONE',  ( 44.81606138205700063, -21.15876147765404625, 76.30501292736998664 ) ) ;
#3584=EDGE_CURVE ( 'NONE', #13207, #10501, #2799, .T. ) ;
#3588=ORIENTED_EDGE ( 'NONE', *, *, #3273, .F. ) ;
#3591=CIRCLE ( 'NONE', #15935, 0.7500000000000006661 ) ;
#3592=CARTESIAN_POINT ( 'NONE',  ( 41.14099152588522657, 40.39281886181299797, 84.30501292736984453 ) ) ;
#3596=CARTESIAN_POINT ( 'NONE',  ( 44.81606138205700063, -33.05876147765410167, 70.30501292737000085 ) ) ;
#3601=DIRECTION ( 'NONE',  ( 1.000000000000000000, 0.000000000000000000, 0.000000000000000000 ) ) ;
#3634=VERTEX_POINT ( 'NONE', #11328 ) ;
#3651=ORIENTED_EDGE ( 'NONE', *, *, #15292, .T. ) ;
#3656=CARTESIAN_POINT ( 'NONE',  ( 38.41621794735363693, -36.60729675983900222, 83.30501292737011454 ) ) ;
#3668=AXIS2_PLACEMENT_3D ( 'NONE', #21864, #12088, #1884 ) ;
#3693=CARTESIAN_POINT ( 'NONE',  ( 31.81606138205700418, 0.1601050959395486362, 68.80395113470939350 ) ) ;
#3702=EDGE_LOOP ( 'NONE', ( #3708, #18334, #10522, #3953 ) ) ;
#3708=ORIENTED_EDGE ( 'NONE', *, *, #11770, .F. ) ;
#3710=CARTESIAN_POINT ( 'NONE',  ( 35.14099152588523367, -10.60718113818700026, 93.30501292736998664 ) ) ;
#3720=ADVANCED_FACE ( 'NONE', ( #17750 ), #21737, .T. ) ;
#3724=DIRECTION ( 'NONE',  ( 0.000000000000000000, 0.000000000000000000, 1.000000000000000000 ) ) ;
#3733=ORIENTED_EDGE ( 'NONE', *, *, #1251, .T. ) ;
#3751=CARTESIAN_POINT ( 'NONE',  ( 35.64099152588522657, 1.392818861812999964, 83.30501292736997243 ) ) ;
#3755=DIRECTION ( 'NONE',  ( 1.734723475976804876E-16, 3.491481338843135327E-15, 1.000000000000000000 ) ) ;
#3761=ADVANCED_FACE ( 'NONE', ( #14262 ), #15928, .F. ) ;
#3764=VECTOR ( 'NONE', #17293, 1000.000000000000000 ) ;
#3773=EDGE_CURVE ( 'NONE', #194, #22820, #24037, .T. ) ;
#3775=CARTESIAN_POINT ( 'NONE',  ( 31.81606138205700418, -27.70293563151089700, 74.66612024218476051 ) ) ;
#3776=CARTESIAN_POINT ( 'NONE',  ( 44.06606138205700063, -26.74044063519535186, 83.30501292737007191 ) ) ;
#3790=FACE_OUTER_BOUND ( 'NONE', #12242, .T. ) ;
#3792=CARTESIAN_POINT ( 'NONE',  ( 38.31606138205700063, 0.6124887759231013584, 81.37823623207334833 ) ) ;
#3799=ORIENTED_EDGE ( 'NONE', *, *, #6026, .T. ) ;
#3802=ADVANCED_FACE ( 'NONE', ( #21613 ), #14012, .T. ) ;
#3809=CARTESIAN_POINT ( 'NONE',  ( 44.81606138205700063, -34.55876147765410167, 70.30501292737000085 ) ) ;
#3810=VECTOR ( 'NONE', #24922, 1000.000000000000000 ) ;
#3815=DIRECTION ( 'NONE',  ( -1.734723475976804876E-16, -3.491481338843135327E-15, -1.000000000000000000 ) ) ;
#3821=VERTEX_POINT ( 'NONE', #13648 ) ;
#3822=DIRECTION ( 'NONE',  ( -1.000000000000000000, -1.734723475976804876E-16, 1.734723475976814737E-16 ) ) ;
#3832=ORIENTED_EDGE ( 'NONE', *, *, #22638, .T. ) ;
#3834=CARTESIAN_POINT ( 'NONE',  ( 35.14099152588522657, -10.60718113818700026, 83.30501292737001506 ) ) ;
#3836=EDGE_LOOP ( 'NONE', ( #2495, #14993, #21778, #3968 ) ) ;
#3838=( GEOMETRIC_REPRESENTATION_CONTEXT ( 3 ) GLOBAL_UNCERTAINTY_ASSIGNED_CONTEXT ( ( #12881 ) ) GLOBAL_UNIT_ASSIGNED_CONTEXT ( ( #19182, #25209, #13515 ) ) REPRESENTATION_CONTEXT ( 'NONE', 'WORKASPACE' ) );
#3840=CARTESIAN_POINT ( 'NONE',  ( 32.56606138205700773, 43.04446929126255128, 81.37823623207322044 ) ) ;
#3859=AXIS2_PLACEMENT_3D ( 'NONE', #2045, #3860, #19573 ) ;
#3860=DIRECTION ( 'NONE',  ( 1.000000000000000000, 1.734723475976799945E-16, -1.734723475976814737E-16 ) ) ;
#3863=VERTEX_POINT ( 'NONE', #23045 ) ;
#3868=ORIENTED_EDGE ( 'NONE', *, *, #12339, .F. ) ;
#3881=CARTESIAN_POINT ( 'NONE',  ( 45.81606138205700063, 40.39281886181299797, 82.55501292736983032 ) ) ;
#3889=EDGE_CURVE ( 'NONE', #4384, #17348, #7469, .T. ) ;
#3891=CARTESIAN_POINT ( 'NONE',  ( 32.56606138205700773, 40.39281886181299797, 82.55501292736983032 ) ) ;
#3897=AXIS2_PLACEMENT_3D ( 'NONE', #5051, #13173, #20777 ) ;
#3899=EDGE_CURVE ( 'NONE', #21678, #1971, #19068, .T. ) ;
#3900=CARTESIAN_POINT ( 'NONE',  ( 44.81606138205700063, -36.30035594811090505, 74.91924054225879104 ) ) ;
#3903=ORIENTED_EDGE ( 'NONE', *, *, #3889, .T. ) ;
#3914=CARTESIAN_POINT ( 'NONE',  ( 44.81606138205700063, 31.19260082947834078, 104.9690409559304101 ) ) ;
#3917=DIRECTION ( 'NONE',  ( 0.2503287245161955887, 0.9681609007195522976, -3.423740829372836395E-15 ) ) ;
#3923=ORIENTED_EDGE ( 'NONE', *, *, #19323, .T. ) ;
#3925=FACE_OUTER_BOUND ( 'NONE', #4632, .T. ) ;
#3926=PLANE ( 'NONE',  #16328 ) ;
#3933=DIRECTION ( 'NONE',  ( -1.301042606982603842E-16, 0.000000000000000000, -1.000000000000000000 ) ) ;
#3937=DIRECTION ( 'NONE',  ( 1.000000000000000000, 4.336808689942014655E-17, -1.734723475976809806E-16 ) ) ;
#3939=ORIENTED_EDGE ( 'NONE', *, *, #13826, .T. ) ;
#3947=ORIENTED_EDGE ( 'NONE', *, *, #13341, .T. ) ;
#3953=ORIENTED_EDGE ( 'NONE', *, *, #11175, .F. ) ;
#3954=ORIENTED_EDGE ( 'NONE', *, *, #12871, .F. ) ;
#3958=EDGE_CURVE ( 'NONE', #15554, #13947, #17136, .T. ) ;
#3968=ORIENTED_EDGE ( 'NONE', *, *, #24575, .T. ) ;
#3974=ORIENTED_EDGE ( 'NONE', *, *, #11326, .T. ) ;
#3984=VECTOR ( 'NONE', #12050, 1000.000000000000000 ) ;
#4001=LINE ( 'NONE', #11751, #4946 ) ;
#4005=AXIS2_PLACEMENT_3D ( 'NONE', #19163, #17234, #25059 ) ;
#4008=FACE_OUTER_BOUND ( 'NONE', #21018, .T. ) ;
#4009=DIRECTION ( 'NONE',  ( -1.000000000000000000, 6.018531076210140067E-31, 1.734723475976804876E-16 ) ) ;
#4025=ADVANCED_FACE ( 'NONE', ( #6919 ), #24421, .F. ) ;
#4046=CARTESIAN_POINT ( 'NONE',  ( 31.81606138205700418, -34.55876147765410167, 70.30501292737000085 ) ) ;
#4050=EDGE_CURVE ( 'NONE', #7938, #23852, #11309, .T. ) ;
#4061=ORIENTED_EDGE ( 'NONE', *, *, #2467, .F. ) ;
#4066=ORIENTED_EDGE ( 'NONE', *, *, #4372, .T. ) ;
#4067=EDGE_CURVE ( 'NONE', #3225, #10628, #17265, .T. ) ;
#4073=ORIENTED_EDGE ( 'NONE', *, *, #15725, .F. ) ;
#4082=EDGE_CURVE ( 'NONE', #21871, #1577, #14643, .T. ) ;
#4101=DIRECTION ( 'NONE',  ( -1.734723475976814737E-16, 1.000000000000000000, -3.491481338843135327E-15 ) ) ;
#4104=PRODUCT_DEFINITION_CONTEXT ( 'detailed design', #5680, 'design' ) ;
#4111=CIRCLE ( 'NONE', #10303, 10.00000000000000178 ) ;
#4112=VERTEX_POINT ( 'NONE', #23007 ) ;
#4132=VECTOR ( 'NONE', #24496, 1000.000000000000000 ) ;
#4140=PLANE ( 'NONE',  #10202 ) ;
#4144=PLANE ( 'NONE',  #7558 ) ;
#4165=LINE ( 'NONE', #401, #3289 ) ;
#4166=DIRECTION ( 'NONE',  ( -1.000000000000000000, 0.000000000000000000, 0.000000000000000000 ) ) ;
#4171=ORIENTED_EDGE ( 'NONE', *, *, #14095, .T. ) ;
#4179=ORIENTED_EDGE ( 'NONE', *, *, #3584, .F. ) ;
#4184=CARTESIAN_POINT ( 'NONE',  ( 31.81606138205700418, -38.55876147765429351, 66.30501292737328356 ) ) ;
#4185=ORIENTED_EDGE ( 'NONE', *, *, #21470, .F. ) ;
#4219=CARTESIAN_POINT ( 'NONE',  ( 44.81606138205700063, 39.39281886181299797, 81.75501292736983316 ) ) ;
#4223=DIRECTION ( 'NONE',  ( -1.734723475976804876E-16, -3.491481338843135327E-15, -1.000000000000000000 ) ) ;
#4224=ORIENTED_EDGE ( 'NONE', *, *, #23336, .F. ) ;
#4235=LINE ( 'NONE', #3840, #19006 ) ;
#4244=AXIS2_PLACEMENT_3D ( 'NONE', #8176, #14099, #23997 ) ;
#4247=VECTOR ( 'NONE', #24512, 1000.000000000000000 ) ;
#4268=VERTEX_POINT ( 'NONE', #8703 ) ;
#4299=CARTESIAN_POINT ( 'NONE',  ( 40.64099152588522657, -1.357181138186998925, 80.05501292737000085 ) ) ;
#4303=LINE ( 'NONE', #280, #17492 ) ;
#4311=ORIENTED_EDGE ( 'NONE', *, *, #8829, .F. ) ;
#4314=CARTESIAN_POINT ( 'NONE',  ( 30.81606138205700418, 1.142818861812999742, 83.30501292736997243 ) ) ;
#4317=CARTESIAN_POINT ( 'NONE',  ( 35.64099152588522657, -9.607181138187000258, 80.05501292737000085 ) ) ;
#4319=ORIENTED_EDGE ( 'NONE', *, *, #6414, .T. ) ;
#4320=DIRECTION ( 'NONE',  ( -1.734723475976804876E-16, 1.000000000000000000, 0.000000000000000000 ) ) ;
#4322=PLANE ( 'NONE',  #6993 ) ;
#4327=ORIENTED_EDGE ( 'NONE', *, *, #9499, .T. ) ;
#4335=VERTEX_POINT ( 'NONE', #21966 ) ;
#4341=DIRECTION ( 'NONE',  ( -1.000000000000000000, 0.000000000000000000, 0.000000000000000000 ) ) ;
#4350=DIRECTION ( 'NONE',  ( -1.000000000000000000, -2.065146995210479765E-16, 1.734723475976814737E-16 ) ) ;
#4353=DIRECTION ( 'NONE',  ( -1.000000000000000000, -1.734723475976804876E-16, 1.734723475976814737E-16 ) ) ;
#4372=EDGE_CURVE ( 'NONE', #10140, #17540, #5209, .T. ) ;
#4375=DIRECTION ( 'NONE',  ( 0.000000000000000000, 0.000000000000000000, 1.000000000000000000 ) ) ;
#4379=EDGE_CURVE ( 'NONE', #19007, #18511, #14995, .T. ) ;
#4380=ORIENTED_EDGE ( 'NONE', *, *, #8306, .T. ) ;
#4384=VERTEX_POINT ( 'NONE', #18736 ) ;
#4392=CARTESIAN_POINT ( 'NONE',  ( 41.14099152588523367, -10.60718113818700026, 93.30501292736998664 ) ) ;
#4393=ORIENTED_EDGE ( 'NONE', *, *, #25139, .T. ) ;
#4408=PLANE ( 'NONE',  #19723 ) ;
#4418=DIRECTION ( 'NONE',  ( 0.000000000000000000, -1.000000000000000000, 3.304235192336775512E-15 ) ) ;
#4428=ADVANCED_FACE ( 'NONE', ( #22973 ), #9340, .T. ) ;
#4432=VERTEX_POINT ( 'NONE', #6879 ) ;
#4439=LINE ( 'NONE', #4317, #10021 ) ;
#4460=DIRECTION ( 'NONE',  ( 1.000000000000000000, -6.018531076210110289E-31, -1.734723475976804876E-16 ) ) ;
#4463=ADVANCED_FACE ( 'NONE', ( #2870, #942 ), #16672, .F. ) ;
#4481=LINE ( 'NONE', #17888, #20907 ) ;
#4482=DIRECTION ( 'NONE',  ( -1.734723475976804876E-16, -3.491481338843135327E-15, -1.000000000000000000 ) ) ;
#4483=ORIENTED_EDGE ( 'NONE', *, *, #13189, .T. ) ;
#4487=VERTEX_POINT ( 'NONE', #19363 ) ;
#4506=VERTEX_POINT ( 'NONE', #5971 ) ;
#4509=VECTOR ( 'NONE', #7727, 1000.000000000000000 ) ;
#4516=EDGE_CURVE ( 'NONE', #3821, #131, #19612, .T. ) ;
#4519=FACE_OUTER_BOUND ( 'NONE', #11346, .T. ) ;
#4542=CARTESIAN_POINT ( 'NONE',  ( 30.81606138205700418, 40.39281886181299797, 66.30501292737000085 ) ) ;
#4548=DIRECTION ( 'NONE',  ( 1.000000000000000000, 2.065146995210479765E-16, -1.734723475976814737E-16 ) ) ;
#4549=DIRECTION ( 'NONE',  ( 0.000000000000000000, -1.000000000000000000, 0.000000000000000000 ) ) ;
#4554=CARTESIAN_POINT ( 'NONE',  ( 38.41621794735363693, -36.60729675983900222, 83.30501292737011454 ) ) ;
#4557=EDGE_CURVE ( 'NONE', #9294, #2245, #8036, .T. ) ;
#4573=CARTESIAN_POINT ( 'NONE',  ( 44.81606138205700063, 34.87886987267150118, 80.75501292736984738 ) ) ;
#4576=ORIENTED_EDGE ( 'NONE', *, *, #15465, .T. ) ;
#4580=ORIENTED_EDGE ( 'NONE', *, *, #7183, .T. ) ;
#4593=ORIENTED_EDGE ( 'NONE', *, *, #2921, .T. ) ;
#4598=DIRECTION ( 'NONE',  ( 1.510383499235849534E-16, 0.1218693434051499741, 0.9925461516413217611 ) ) ;
#4600=DIRECTION ( 'NONE',  ( 1.000000000000000000, 1.734723475976804876E-16, -1.734723475976814737E-16 ) ) ;
#4602=LINE ( 'NONE', #18011, #14789 ) ;
#4603=CARTESIAN_POINT ( 'NONE',  ( 30.81606138205700418, 1.392818861812999964, 84.30501292737000085 ) ) ;
#4604=EDGE_CURVE ( 'NONE', #7039, #13966, #13821, .T. ) ;
#4614=DIRECTION ( 'NONE',  ( 1.000000000000000000, 0.000000000000000000, -1.734723475976814737E-16 ) ) ;
#4618=ADVANCED_FACE ( 'NONE', ( #17443 ), #21679, .T. ) ;
#4623=CARTESIAN_POINT ( 'NONE',  ( 35.64099152588523367, 1.142818861812999742, 93.30501292736998664 ) ) ;
#4625=VECTOR ( 'NONE', #22753, 1000.000000000000000 ) ;
#4632=EDGE_LOOP ( 'NONE', ( #6317, #8991, #6559, #306 ) ) ;
#4642=CARTESIAN_POINT ( 'NONE',  ( 45.81606138205700063, -33.05876147765410167, 70.30501292737000085 ) ) ;
#4655=DIRECTION ( 'NONE',  ( -1.000000000000000000, 6.018531076210130433E-31, 1.734723475976804876E-16 ) ) ;
#4663=VECTOR ( 'NONE', #23361, 1000.000000000000000 ) ;
#4668=CARTESIAN_POINT ( 'NONE',  ( 31.81606138205700418, -3.831401139557048197, 80.75501292737000369 ) ) ;
#4678=CIRCLE ( 'NONE', #21559, 3.000000000000002665 ) ;
#4681=CARTESIAN_POINT ( 'NONE',  ( 34.56606138205700773, 45.04446929126260102, 82.37823623207320622 ) ) ;
#4684=DIRECTION ( 'NONE',  ( -1.734723475976814737E-16, 0.000000000000000000, -1.000000000000000000 ) ) ;
#4689=ADVANCED_FACE ( 'NONE', ( #21934 ), #10600, .F. ) ;
#4691=DIRECTION ( 'NONE',  ( 0.000000000000000000, 0.000000000000000000, -1.000000000000000000 ) ) ;
#4700=STYLED_ITEM ( 'NONE', ( #18368 ), #16726 ) ;
#4722=CARTESIAN_POINT ( 'NONE',  ( 44.06606138205700063, 42.11769259596595560, 81.89079936499673806 ) ) ;
#4724=EDGE_CURVE ( 'NONE', #19809, #4112, #4165, .T. ) ;
#4727=FACE_BOUND ( 'NONE', #15687, .T. ) ;
#4731=DIRECTION ( 'NONE',  ( 8.791731484610113542E-17, -0.9135454576426023099, -0.4067366430757970996 ) ) ;
#4738=ORIENTED_EDGE ( 'NONE', *, *, #21348, .F. ) ;
#4777=CARTESIAN_POINT ( 'NONE',  ( 40.64099152588523367, 1.832818861813001021, 88.30501292736998664 ) ) ;
#4783=VERTEX_POINT ( 'NONE', #20127 ) ;
#4792=DIRECTION ( 'NONE',  ( 0.000000000000000000, 1.000000000000000000, 0.000000000000000000 ) ) ;
#4794=FACE_OUTER_BOUND ( 'NONE', #15839, .T. ) ;
#4818=DIRECTION ( 'NONE',  ( -1.000000000000000000, 6.018531076210110289E-31, 1.734723475976804876E-16 ) ) ;
#4827=EDGE_CURVE ( 'NONE', #20770, #1205, #15876, .T. ) ;
#4831=EDGE_CURVE ( 'NONE', #15469, #12300, #4111, .T. ) ;
#4832=LINE ( 'NONE', #957, #14673 ) ;
#4843=DIRECTION ( 'NONE',  ( 0.000000000000000000, -1.000000000000000000, 3.469446951953611033E-15 ) ) ;
#4858=ORIENTED_EDGE ( 'NONE', *, *, #21536, .T. ) ;
#4859=ORIENTED_EDGE ( 'NONE', *, *, #5796, .F. ) ;
#4870=PLANE ( 'NONE',  #5075 ) ;
#4887=CARTESIAN_POINT ( 'NONE',  ( 30.81606138205700418, 24.50429740018177682, 101.9912164131601457 ) ) ;
#4906=ORIENTED_EDGE ( 'NONE', *, *, #14443, .T. ) ;
#4907=DIRECTION ( 'NONE',  ( 1.000000000000000000, 0.000000000000000000, 0.000000000000000000 ) ) ;
#4922=CARTESIAN_POINT ( 'NONE',  ( 59.50607210797845426, 32.97469880962110267, 83.30501292736985874 ) ) ;
#4946=VECTOR ( 'NONE', #17407, 1000.000000000000114 ) ;
#4948=ORIENTED_EDGE ( 'NONE', *, *, #21348, .T. ) ;
#4950=DIRECTION ( 'NONE',  ( -1.000000000000000000, -1.734723475976804876E-16, 1.734723475976814737E-16 ) ) ;
#4951=FACE_OUTER_BOUND ( 'NONE', #25329, .T. ) ;
#4960=EDGE_LOOP ( 'NONE', ( #9982, #2506, #76, #3173 ) ) ;
#4971=CARTESIAN_POINT ( 'NONE',  ( 30.81606138205700418, -27.70293563151089700, 74.66612024218476051 ) ) ;
#4975=CARTESIAN_POINT ( 'NONE',  ( 32.56606138205700773, 40.92314894770289158, 83.08534301325974525 ) ) ;
#4979=ADVANCED_FACE ( 'NONE', ( #8920 ), #6722, .T. ) ;
#4985=DIRECTION ( 'NONE',  ( 0.000000000000000000, 1.000000000000000000, 0.000000000000000000 ) ) ;
#4989=ORIENTED_EDGE ( 'NONE', *, *, #9675, .T. ) ;
#4993=DIRECTION ( 'NONE',  ( -1.000000000000000000, 0.000000000000000000, 0.000000000000000000 ) ) ;
#5002=LINE ( 'NONE', #24692, #23006 ) ;
#5017=DIRECTION ( 'NONE',  ( -1.000000000000000000, -1.734723475976804876E-16, 1.734723475976814737E-16 ) ) ;
#5025=DIRECTION ( 'NONE',  ( -1.000000000000000000, -1.734723475976804876E-16, 1.734723475976814737E-16 ) ) ;
#5049=ORIENTED_EDGE ( 'NONE', *, *, #3958, .T. ) ;
#5051=CARTESIAN_POINT ( 'NONE',  ( 32.56606138205700773, 43.35512946304240245, 83.12823623207320622 ) ) ;
#5059=CARTESIAN_POINT ( 'NONE',  ( 44.81606138205700063, 40.39281886181299797, 84.30501292736984453 ) ) ;
#5074=CARTESIAN_POINT ( 'NONE',  ( 35.64099152588523367, 1.392818861812999964, 93.30501292736998664 ) ) ;
#5075=AXIS2_PLACEMENT_3D ( 'NONE', #16585, #3182, #1114 ) ;
#5084=VECTOR ( 'NONE', #24243, 1000.000000000000000 ) ;
#5085=LINE ( 'NONE', #12949, #1356 ) ;
#5091=VECTOR ( 'NONE', #14837, 1000.000000000000000 ) ;
#5097=AXIS2_PLACEMENT_3D ( 'NONE', #20522, #2855, #4684 ) ;
#5102=EDGE_LOOP ( 'NONE', ( #15672, #9611, #19295, #19136 ) ) ;
#5107=CARTESIAN_POINT ( 'NONE',  ( 32.56606138205700773, -26.74044063519535186, 83.30501292737007191 ) ) ;
#5108=AXIS2_PLACEMENT_3D ( 'NONE', #21005, #3348, #19194 ) ;
#5117=EDGE_CURVE ( 'NONE', #24557, #14211, #4001, .T. ) ;
#5120=VERTEX_POINT ( 'NONE', #23190 ) ;
#5131=VECTOR ( 'NONE', #2851, 999.9999999999998863 ) ;
#5138=LINE ( 'NONE', #6933, #19653 ) ;
#5140=DIRECTION ( 'NONE',  ( -1.734723475976804876E-16, -3.491481338843135327E-15, -1.000000000000000000 ) ) ;
#5154=CARTESIAN_POINT ( 'NONE',  ( 44.06606138205700063, 40.39281886181299797, 82.55501292736983032 ) ) ;
#5185=DIRECTION ( 'NONE',  ( 1.000000000000000000, 3.197344634236645231E-31, -1.734723475976814737E-16 ) ) ;
#5188=DIRECTION ( 'NONE',  ( -1.000000000000000000, -1.734723475976804876E-16, 1.734723475976814737E-16 ) ) ;
#5197=CARTESIAN_POINT ( 'NONE',  ( 44.81606138205700063, 34.87886987267150118, 80.75501292736991843 ) ) ;
#5209=LINE ( 'NONE', #22720, #21793 ) ;
#5216=CARTESIAN_POINT ( 'NONE',  ( 44.06606138205700063, 47.04446929126260102, 81.37823623207319201 ) ) ;
#5232=FACE_BOUND ( 'NONE', #5527, .T. ) ;
#5248=FACE_OUTER_BOUND ( 'NONE', #17877, .T. ) ;
#5255=CARTESIAN_POINT ( 'NONE',  ( 40.64099152588522657, 1.142818861812999742, 82.55501292736997243 ) ) ;
#5272=VECTOR ( 'NONE', #4223, 1000.000000000000000 ) ;
#5274=VERTEX_POINT ( 'NONE', #22149 ) ;
#5284=LINE ( 'NONE', #21506, #14344 ) ;
#5293=AXIS2_PLACEMENT_3D ( 'NONE', #11470, #9918, #25083 ) ;
#5300=ORIENTED_EDGE ( 'NONE', *, *, #16, .F. ) ;
#5302=ORIENTED_EDGE ( 'NONE', *, *, #8885, .F. ) ;
#5310=FACE_OUTER_BOUND ( 'NONE', #21323, .T. ) ;
#5322=DIRECTION ( 'NONE',  ( -1.000000000000000000, 6.018531076210110289E-31, 1.734723475976804876E-16 ) ) ;
#5327=VECTOR ( 'NONE', #21485, 1000.000000000000000 ) ;
#5337=CARTESIAN_POINT ( 'NONE',  ( 32.56606138205700773, -26.74044063519535186, 82.55501292737007191 ) ) ;
#5364=VECTOR ( 'NONE', #8564, 1000.000000000000000 ) ;
#5375=ORIENTED_EDGE ( 'NONE', *, *, #729, .F. ) ;
#5379=LINE ( 'NONE', #17108, #12458 ) ;
#5391=CARTESIAN_POINT ( 'NONE',  ( 44.81606138205700063, 0.1601050959395486362, 68.80395113470939350 ) ) ;
#5401=DIRECTION ( 'NONE',  ( 1.734723475976805122E-16, -1.000000000000000000, 0.000000000000000000 ) ) ;
#5404=ORIENTED_EDGE ( 'NONE', *, *, #14904, .F. ) ;
#5415=CARTESIAN_POINT ( 'NONE',  ( 32.56606138205700773, 40.39281886181299797, 83.30501292736984453 ) ) ;
#5459=DIRECTION ( 'NONE',  ( -1.000000000000000000, 0.000000000000000000, 0.000000000000000000 ) ) ;
#5476=DIRECTION ( 'NONE',  ( 0.000000000000000000, 1.000000000000000000, -4.625929269271481378E-15 ) ) ;
#5477=ADVANCED_FACE ( 'NONE', ( #14667 ), #20738, .F. ) ;
#5488=VECTOR ( 'NONE', #5577, 1000.000000000000000 ) ;
#5496=EDGE_LOOP ( 'NONE', ( #2029, #8955, #17096, #22123 ) ) ;
#5503=CIRCLE ( 'NONE', #8390, 3.999999999999996447 ) ;
#5513=VECTOR ( 'NONE', #3724, 1000.000000000000000 ) ;
#5527=EDGE_LOOP ( 'NONE', ( #16003, #13218 ) ) ;
#5542=DIRECTION ( 'NONE',  ( 4.336808689942074435E-17, -1.000000000000000000, 3.491481338843135327E-15 ) ) ;
#5558=ADVANCED_FACE ( 'NONE', ( #20354 ), #2683, .T. ) ;
#5561=LINE ( 'NONE', #9437, #8963 ) ;
#5562=ORIENTED_EDGE ( 'NONE', *, *, #20361, .T. ) ;
#5563=CARTESIAN_POINT ( 'NONE',  ( 30.81606138205700418, -36.05876147765410877, 70.30501292737000085 ) ) ;
#5577=DIRECTION ( 'NONE',  ( 1.000000000000000000, 1.734723475976804876E-16, -1.734723475976814737E-16 ) ) ;
#5591=ORIENTED_EDGE ( 'NONE', *, *, #3899, .F. ) ;
#5594=ORIENTED_EDGE ( 'NONE', *, *, #12133, .F. ) ;
#5601=FACE_OUTER_BOUND ( 'NONE', #16538, .T. ) ;
#5603=EDGE_CURVE ( 'NONE', #10371, #11274, #16904, .T. ) ;
#5611=CARTESIAN_POINT ( 'NONE',  ( 30.81606138205700418, 40.39281886181299797, 82.55501292736983032 ) ) ;
#5620=ORIENTED_EDGE ( 'NONE', *, *, #11152, .T. ) ;
#5650=CARTESIAN_POINT ( 'NONE',  ( 30.81606138205700418, -39.60718113818700203, 83.30501292737011454 ) ) ;
#5654=EDGE_LOOP ( 'NONE', ( #19066, #1346, #20050, #20405 ) ) ;
#5665=EDGE_LOOP ( 'NONE', ( #4858, #11044, #3195, #11714 ) ) ;
#5667=EDGE_CURVE ( 'NONE', #4384, #18087, #11695, .T. ) ;
#5680=APPLICATION_CONTEXT ( 'automotive_design' ) ;
#5683=DIRECTION ( 'NONE',  ( -2.478176394252580155E-16, 0.000000000000000000, -1.000000000000000000 ) ) ;
#5686=DIRECTION ( 'NONE',  ( -1.000000000000000000, 6.018531076210110289E-31, 1.734723475976804876E-16 ) ) ;
#5692=VECTOR ( 'NONE', #332, 1000.000000000000000 ) ;
#5713=AXIS2_PLACEMENT_3D ( 'NONE', #12688, #806, #4691 ) ;
#5739=EDGE_LOOP ( 'NONE', ( #14750, #6008, #17895, #11523 ) ) ;
#5747=ORIENTED_EDGE ( 'NONE', *, *, #22486, .T. ) ;
#5751=DIRECTION ( 'NONE',  ( 1.000000000000000000, 0.000000000000000000, 0.000000000000000000 ) ) ;
#5759=ORIENTED_EDGE ( 'NONE', *, *, #9428, .T. ) ;
#5760=CARTESIAN_POINT ( 'NONE',  ( 31.81606138205700418, -38.55876147765410167, 70.30501292737011454 ) ) ;
#5765=VECTOR ( 'NONE', #9683, 1000.000000000000000 ) ;
#5772=ORIENTED_EDGE ( 'NONE', *, *, #2921, .F. ) ;
#5774=EDGE_LOOP ( 'NONE', ( #10503, #3832, #119, #5772 ) ) ;
#5779=EDGE_CURVE ( 'NONE', #14211, #15541, #8580, .T. ) ;
#5780=LINE ( 'NONE', #9780, #14072 ) ;
#5785=CARTESIAN_POINT ( 'NONE',  ( 38.41621794735363693, -38.10729675983899511, 84.30501292737011454 ) ) ;
#5796=EDGE_CURVE ( 'NONE', #2551, #22728, #23874, .T. ) ;
#5806=VERTEX_POINT ( 'NONE', #22474 ) ;
#5817=ORIENTED_EDGE ( 'NONE', *, *, #23741, .F. ) ;
#5819=DIRECTION ( 'NONE',  ( 1.000000000000000000, 2.168404344971005170E-16, -1.734723475976814737E-16 ) ) ;
#5825=LINE ( 'NONE', #9325, #2732 ) ;
#5838=ORIENTED_EDGE ( 'NONE', *, *, #7644, .F. ) ;
#5846=EDGE_LOOP ( 'NONE', ( #20851, #4576, #24705, #14519 ) ) ;
#5851=CARTESIAN_POINT ( 'NONE',  ( 31.81606138205700418, 34.87886987267149408, 80.75501292736984738 ) ) ;
#5856=AXIS2_PLACEMENT_3D ( 'NONE', #6674, #14166, #22014 ) ;
#5859=CARTESIAN_POINT ( 'NONE',  ( 31.81606138205700418, -26.74044063519544778, 66.30501292737000085 ) ) ;
#5875=CARTESIAN_POINT ( 'NONE',  ( 34.56606138205700773, 47.04446929126254417, 81.37823623207319201 ) ) ;
#5878=EDGE_LOOP ( 'NONE', ( #11010, #19176, #7935, #24324 ) ) ;
#5899=DIRECTION ( 'NONE',  ( -1.734723475976814737E-16, 1.000000000000000000, -3.491481338843135327E-15 ) ) ;
#5913=ORIENTED_EDGE ( 'NONE', *, *, #21686, .T. ) ;
#5916=VECTOR ( 'NONE', #13547, 1000.000000000000000 ) ;
#5938=VERTEX_POINT ( 'NONE', #17191 ) ;
#5945=DIRECTION ( 'NONE',  ( -7.292888252353849301E-16, 0.000000000000000000, 1.000000000000000000 ) ) ;
#5971=CARTESIAN_POINT ( 'NONE',  ( 44.81606138205700063, -31.45856502260510013, 77.07494475056050476 ) ) ;
#5974=ORIENTED_EDGE ( 'NONE', *, *, #22310, .F. ) ;
#5976=LINE ( 'NONE', #13956, #16211 ) ;
#5981=CARTESIAN_POINT ( 'NONE',  ( 59.50607210797845426, 32.97469880962110267, 84.30501292736985874 ) ) ;
#5996=ORIENTED_EDGE ( 'NONE', *, *, #24590, .T. ) ;
#5998=DIRECTION ( 'NONE',  ( -1.734723475976804876E-16, -3.491481338843135327E-15, -1.000000000000000000 ) ) ;
#6002=ORIENTED_EDGE ( 'NONE', *, *, #9428, .F. ) ;
#6003=ORIENTED_EDGE ( 'NONE', *, *, #24575, .F. ) ;
#6008=ORIENTED_EDGE ( 'NONE', *, *, #18535, .F. ) ;
#6011=ORIENTED_EDGE ( 'NONE', *, *, #7366, .T. ) ;
#6021=CYLINDRICAL_SURFACE ( 'NONE', #19673, 4.000000000000000000 ) ;
#6026=EDGE_CURVE ( 'NONE', #5120, #25303, #14864, .T. ) ;
#6028=CARTESIAN_POINT ( 'NONE',  ( 31.81606138205700418, 39.39281886181299797, 81.75501292736984738 ) ) ;
#6050=AXIS2_PLACEMENT_3D ( 'NONE', #8915, #22301, #12912 ) ;
#6067=CIRCLE ( 'NONE', #12660, 1.750000000000001554 ) ;
#6082=DIRECTION ( 'NONE',  ( -1.000000000000000000, 0.000000000000000000, 0.000000000000000000 ) ) ;
#6083=EDGE_CURVE ( 'NONE', #6422, #12591, #5976, .T. ) ;
#6106=DIRECTION ( 'NONE',  ( 1.000000000000000000, 1.734723475976804876E-16, -1.734723475976814737E-16 ) ) ;
#6120=ADVANCED_FACE ( 'NONE', ( #19751 ), #25143, .F. ) ;
#6140=CYLINDRICAL_SURFACE ( 'NONE', #1317, 0.7500000000000006661 ) ;
#6149=EDGE_CURVE ( 'NONE', #6360, #4384, #31, .T. ) ;
#6156=CARTESIAN_POINT ( 'NONE',  ( 30.81606138205700418, 34.87886987267149408, 66.30501292737000085 ) ) ;
#6178=DIRECTION ( 'NONE',  ( 1.000000000000000000, 0.000000000000000000, 0.000000000000000000 ) ) ;
#6189=DIRECTION ( 'NONE',  ( 1.000000000000000000, 1.734723475976804876E-16, -1.734723475976814737E-16 ) ) ;
#6191=ORIENTED_EDGE ( 'NONE', *, *, #18853, .F. ) ;
#6210=DIRECTION ( 'NONE',  ( -6.489379976170840313E-31, 1.000000000000000000, -3.491481338843135327E-15 ) ) ;
#6228=CARTESIAN_POINT ( 'NONE',  ( 40.64099152588522657, 1.392818861812999964, 84.30501292737000085 ) ) ;
#6234=DIRECTION ( 'NONE',  ( -1.000000000000000000, -1.734723475976804876E-16, 1.734723475976814737E-16 ) ) ;
#6249=ORIENTED_EDGE ( 'NONE', *, *, #13341, .F. ) ;
#6269=EDGE_CURVE ( 'NONE', #19362, #16440, #581, .T. ) ;
#6270=VERTEX_POINT ( 'NONE', #22190 ) ;
#6271=ORIENTED_EDGE ( 'NONE', *, *, #3529, .T. ) ;
#6273=EDGE_CURVE ( 'NONE', #7938, #24390, #8290, .T. ) ;
#6278=CARTESIAN_POINT ( 'NONE',  ( 35.64099152588523367, -1.357181138186998925, 88.30501292736998664 ) ) ;
#6282=EDGE_CURVE ( 'NONE', #16594, #16761, #23983, .T. ) ;
#6287=FACE_OUTER_BOUND ( 'NONE', #19389, .T. ) ;
#6288=ORIENTED_EDGE ( 'NONE', *, *, #22314, .T. ) ;
#6299=AXIS2_PLACEMENT_3D ( 'NONE', #15920, #20265, #2602 ) ;
#6317=ORIENTED_EDGE ( 'NONE', *, *, #20599, .F. ) ;
#6322=EDGE_CURVE ( 'NONE', #12591, #194, #4303, .T. ) ;
#6360=VERTEX_POINT ( 'NONE', #6228 ) ;
#6361=ORIENTED_EDGE ( 'NONE', *, *, #11620, .T. ) ;
#6377=CIRCLE ( 'NONE', #3067, 0.7500000000000006661 ) ;
#6403=ORIENTED_EDGE ( 'NONE', *, *, #7196, .F. ) ;
#6406=ORIENTED_EDGE ( 'NONE', *, *, #22491, .F. ) ;
#6411=CARTESIAN_POINT ( 'NONE',  ( 31.81606138205700418, -38.55876147765410167, 72.21586839016146087 ) ) ;
#6414=EDGE_CURVE ( 'NONE', #12560, #21390, #21192, .T. ) ;
#6422=VERTEX_POINT ( 'NONE', #8805 ) ;
#6450=DIRECTION ( 'NONE',  ( -1.734723475976814737E-16, 1.000000000000000000, -3.491481338843135327E-15 ) ) ;
#6458=ADVANCED_FACE ( 'NONE', ( #5310 ), #10980, .F. ) ;
#6478=CARTESIAN_POINT ( 'NONE',  ( 45.81606138205700063, 34.87886987267150118, 78.19668729537065133 ) ) ;
#6483=DIRECTION ( 'NONE',  ( -1.000000000000000000, -1.734723475976804876E-16, 1.734723475976814737E-16 ) ) ;
#6485=ADVANCED_FACE ( 'NONE', ( #21027 ), #23068, .F. ) ;
#6502=VERTEX_POINT ( 'NONE', #6850 ) ;
#6503=AXIS2_PLACEMENT_3D ( 'NONE', #6028, #14143, #8471 ) ;
#6510=ORIENTED_EDGE ( 'NONE', *, *, #18197, .F. ) ;
#6524=LINE ( 'NONE', #6278, #23126 ) ;
#6549=DIRECTION ( 'NONE',  ( 1.000000000000000000, 2.168404344971010101E-16, -1.734723475976814737E-16 ) ) ;
#6558=CARTESIAN_POINT ( 'NONE',  ( 44.81606138205700063, 40.39281886181299797, 82.55501292736983032 ) ) ;
#6559=ORIENTED_EDGE ( 'NONE', *, *, #11868, .T. ) ;
#6569=PLANE ( 'NONE',  #8382 ) ;
#6572=DIRECTION ( 'NONE',  ( 0.000000000000000000, 1.000000000000000000, 0.000000000000000000 ) ) ;
#6579=ADVANCED_FACE ( 'NONE', ( #1548 ), #15851, .F. ) ;
#6592=LINE ( 'NONE', #10470, #3171 ) ;
#6596=ORIENTED_EDGE ( 'NONE', *, *, #16991, .T. ) ;
#6609=DIRECTION ( 'NONE',  ( 2.453269466693404537E-16, -0.7071067811865489050, 0.7071067811865460184 ) ) ;
#6611=PLANE ( 'NONE',  #5097 ) ;
#6612=CARTESIAN_POINT ( 'NONE',  ( 44.06606138205700063, 42.82479937715250173, 82.59790614618329130 ) ) ;
#6638=( NAMED_UNIT ( * ) PLANE_ANGLE_UNIT ( ) SI_UNIT ( $, .RADIAN. ) );
#6639=DIRECTION ( 'NONE',  ( 2.753529326947312927E-16, -1.000000000000000000, 3.304235192336775512E-15 ) ) ;
#6649=CARTESIAN_POINT ( 'NONE',  ( 30.81606138205700418, -34.55876147765410167, 70.30501292737000085 ) ) ;
#6659=ADVANCED_FACE ( 'NONE', ( #4008 ), #2063, .T. ) ;
#6661=VERTEX_POINT ( 'NONE', #5563 ) ;
#6664=CARTESIAN_POINT ( 'NONE',  ( 17.31606138205699708, 42.46194149498198556, 81.44836866983821722 ) ) ;
#6674=CARTESIAN_POINT ( 'NONE',  ( 38.41621794735363693, -36.60729675983900222, 83.30501292737011454 ) ) ;
#6677=CARTESIAN_POINT ( 'NONE',  ( 38.41621794735363693, -36.60729675983900222, 83.30501292737011454 ) ) ;
#6693=CYLINDRICAL_SURFACE ( 'NONE', #19908, 0.7500000000000006661 ) ;
#6696=ORIENTED_EDGE ( 'NONE', *, *, #3889, .F. ) ;
#6701=CIRCLE ( 'NONE', #19462, 0.7500000000000006661 ) ;
#6714=EDGE_CURVE ( 'NONE', #10641, #22820, #15470, .T. ) ;
#6715=FACE_OUTER_BOUND ( 'NONE', #9972, .T. ) ;
#6717=AXIS2_PLACEMENT_3D ( 'NONE', #3282, #15509, #11292 ) ;
#6722=CYLINDRICAL_SURFACE ( 'NONE', #15647, 1.750000000000001554 ) ;
#6734=CIRCLE ( 'NONE', #19073, 1.000000000000000888 ) ;
#6760=CARTESIAN_POINT ( 'NONE',  ( 30.81606138205700418, -34.55876147765410167, 70.30501292737000085 ) ) ;
#6772=CARTESIAN_POINT ( 'NONE',  ( 38.41621794735363693, -38.10729675983899511, 83.30501292737011454 ) ) ;
#6779=PLANE ( 'NONE',  #20708 ) ;
#6806=AXIS2_PLACEMENT_3D ( 'NONE', #14430, #21784, #8258 ) ;
#6807=EDGE_CURVE ( 'NONE', #7351, #18272, #20226, .T. ) ;
#6809=ADVANCED_FACE ( 'NONE', ( #22032, #10447 ), #13928, .T. ) ;
#6812=EDGE_CURVE ( 'NONE', #10765, #18894, #10915, .T. ) ;
#6822=DIRECTION ( 'NONE',  ( -1.000000000000000000, -1.734723475976799945E-16, 1.734723475976814737E-16 ) ) ;
#6827=ORIENTED_EDGE ( 'NONE', *, *, #128, .F. ) ;
#6834=FACE_OUTER_BOUND ( 'NONE', #11735, .T. ) ;
#6843=ORIENTED_EDGE ( 'NONE', *, *, #2982, .F. ) ;
#6850=CARTESIAN_POINT ( 'NONE',  ( 35.14099152588522657, -10.60718113818700026, 84.30501292737000085 ) ) ;
#6862=CARTESIAN_POINT ( 'NONE',  ( 44.81606138205700063, 40.39281886181299797, 66.30501292737000085 ) ) ;
#6870=CARTESIAN_POINT ( 'NONE',  ( 35.52536905565747105, -37.40916500673439771, 84.30501292737011454 ) ) ;
#6878=ORIENTED_EDGE ( 'NONE', *, *, #1686, .F. ) ;
#6879=CARTESIAN_POINT ( 'NONE',  ( 44.81606138205700063, -36.30035594811090505, 74.91924054225879104 ) ) ;
#6887=ORIENTED_EDGE ( 'NONE', *, *, #11175, .T. ) ;
#6891=AXIS2_PLACEMENT_3D ( 'NONE', #3891, #11765, #19599 ) ;
#6892=AXIS2_PLACEMENT_3D ( 'NONE', #1115, #857, #9004 ) ;
#6898=EDGE_LOOP ( 'NONE', ( #19926, #4483, #19609, #20947 ) ) ;
#6899=DIRECTION ( 'NONE',  ( 0.000000000000000000, -1.000000000000000000, 0.000000000000000000 ) ) ;
#6908=CARTESIAN_POINT ( 'NONE',  ( 44.81606138205700063, 40.39281886181299797, 80.75501292736983316 ) ) ;
#6915=DIRECTION ( 'NONE',  ( 0.000000000000000000, -1.000000000000000000, 3.491481338843135327E-15 ) ) ;
#6919=FACE_OUTER_BOUND ( 'NONE', #10445, .T. ) ;
#6927=PLANE ( 'NONE',  #16957 ) ;
#6931=CIRCLE ( 'NONE', #13120, 4.000000000000003553 ) ;
#6933=CARTESIAN_POINT ( 'NONE',  ( 30.81606138205700418, 40.39281886181299797, 83.30501292736984453 ) ) ;
#6942=ORIENTED_EDGE ( 'NONE', *, *, #4082, .T. ) ;
#6950=EDGE_CURVE ( 'NONE', #10501, #18087, #8770, .T. ) ;
#6962=DIRECTION ( 'NONE',  ( 1.000000000000000000, -6.018531076210131309E-31, -1.734723475976804876E-16 ) ) ;
#6967=VECTOR ( 'NONE', #19309, 1000.000000000000000 ) ;
#6973=VECTOR ( 'NONE', #464, 1000.000000000000000 ) ;
#6979=ORIENTED_EDGE ( 'NONE', *, *, #20058, .F. ) ;
#6991=DIRECTION ( 'NONE',  ( 0.000000000000000000, 0.000000000000000000, -1.000000000000000000 ) ) ;
#6993=AXIS2_PLACEMENT_3D ( 'NONE', #13849, #9863, #3933 ) ;
#6996=CARTESIAN_POINT ( 'NONE',  ( 45.81606138205700063, -26.97987052895604876, 80.55501292737007191 ) ) ;
#7011=VECTOR ( 'NONE', #6189, 1000.000000000000000 ) ;
#7014=ORIENTED_EDGE ( 'NONE', *, *, #14823, .T. ) ;
#7026=DIRECTION ( 'NONE',  ( 1.000000000000000000, 1.734723475976805122E-16, 0.000000000000000000 ) ) ;
#7030=DIRECTION ( 'NONE',  ( 0.000000000000000000, -1.000000000000000000, 3.469446951953611033E-15 ) ) ;
#7033=LINE ( 'NONE', #836, #18864 ) ;
#7039=VERTEX_POINT ( 'NONE', #11342 ) ;
#7040=ORIENTED_EDGE ( 'NONE', *, *, #18094, .F. ) ;
#7053=EDGE_CURVE ( 'NONE', #21433, #21711, #22029, .T. ) ;
#7097=EDGE_CURVE ( 'NONE', #9294, #19809, #23161, .T. ) ;
#7100=VECTOR ( 'NONE', #24551, 1000.000000000000000 ) ;
#7107=ORIENTED_EDGE ( 'NONE', *, *, #21240, .T. ) ;
#7121=CIRCLE ( 'NONE', #7550, 1.750000000000001554 ) ;
#7130=DIRECTION ( 'NONE',  ( 1.734723475976804876E-16, 3.491481338843135327E-15, 1.000000000000000000 ) ) ;
#7132=ADVANCED_FACE ( 'NONE', ( #25339 ), #11849, .T. ) ;
#7134=VECTOR ( 'NONE', #20429, 1000.000000000000114 ) ;
#7139=EDGE_LOOP ( 'NONE', ( #13609, #9932, #8187, #18299 ) ) ;
#7140=VERTEX_POINT ( 'NONE', #21122 ) ;
#7146=EDGE_LOOP ( 'NONE', ( #10475, #6596, #4580, #12511 ) ) ;
#7147=DIRECTION ( 'NONE',  ( -1.000000000000000000, -1.734723475976804876E-16, 1.734723475976814737E-16 ) ) ;
#7151=VERTEX_POINT ( 'NONE', #7598 ) ;
#7158=ORIENTED_EDGE ( 'NONE', *, *, #15707, .F. ) ;
#7168=VERTEX_POINT ( 'NONE', #15313 ) ;
#7172=CARTESIAN_POINT ( 'NONE',  ( 31.81606138205700418, -11.72563467517899838, 72.98595903681224684 ) ) ;
#7183=EDGE_CURVE ( 'NONE', #22425, #20770, #23418, .T. ) ;
#7191=CARTESIAN_POINT ( 'NONE',  ( 44.06606138205700063, 43.35512946304240245, 81.37823623207320622 ) ) ;
#7195=FACE_OUTER_BOUND ( 'NONE', #8160, .T. ) ;
#7196=EDGE_CURVE ( 'NONE', #10628, #4783, #15825, .T. ) ;
#7199=PLANE ( 'NONE',  #12680 ) ;
#7205=DIRECTION ( 'NONE',  ( 0.000000000000000000, 0.000000000000000000, -1.000000000000000000 ) ) ;
#7236=ORIENTED_EDGE ( 'NONE', *, *, #7644, .T. ) ;
#7238=ORIENTED_EDGE ( 'NONE', *, *, #23339, .F. ) ;
#7254=CYLINDRICAL_SURFACE ( 'NONE', #17601, 1.750000000000001554 ) ;
#7268=ORIENTED_EDGE ( 'NONE', *, *, #2054, .T. ) ;
#7279=DIRECTION ( 'NONE',  ( -1.734723475976804876E-16, -3.491481338843135327E-15, -1.000000000000000000 ) ) ;
#7291=PLANE ( 'NONE',  #19265 ) ;
#7305=VERTEX_POINT ( 'NONE', #10039 ) ;
#7318=VECTOR ( 'NONE', #14090, 1000.000000000000000 ) ;
#7324=VERTEX_POINT ( 'NONE', #225 ) ;
#7330=DIRECTION ( 'NONE',  ( 1.000000000000000000, 1.734723475976804876E-16, -1.734723475976814737E-16 ) ) ;
#7335=ORIENTED_EDGE ( 'NONE', *, *, #13429, .F. ) ;
#7336=CARTESIAN_POINT ( 'NONE',  ( 42.06606138205700063, 45.04446929126260102, 81.37823623207320622 ) ) ;
#7342=CARTESIAN_POINT ( 'NONE',  ( 44.06606138205700063, -26.74044063519535186, 83.30501292737007191 ) ) ;
#7343=CARTESIAN_POINT ( 'NONE',  ( 45.81606138205700063, -26.74044063519535186, 82.50501292737007475 ) ) ;
#7350=AXIS2_PLACEMENT_3D ( 'NONE', #1854, #7673, #25159 ) ;
#7351=VERTEX_POINT ( 'NONE', #1111 ) ;
#7363=VECTOR ( 'NONE', #22815, 1000.000000000000000 ) ;
#7366=EDGE_CURVE ( 'NONE', #13966, #3395, #19439, .T. ) ;
#7408=EDGE_LOOP ( 'NONE', ( #13777, #17459, #22105, #7238 ) ) ;
#7414=ORIENTED_EDGE ( 'NONE', *, *, #14443, .F. ) ;
#7416=DIRECTION ( 'NONE',  ( 9.614242282381077875E-31, 0.7071067811865460184, 0.7071067811865489050 ) ) ;
#7426=EDGE_LOOP ( 'NONE', ( #17029, #16678, #16634, #3323, #7414, #24320 ) ) ;
#7439=DIRECTION ( 'NONE',  ( 0.000000000000000000, -1.000000000000000000, 6.123233995736769734E-17 ) ) ;
#7444=CARTESIAN_POINT ( 'NONE',  ( 30.81606138205700418, -26.97987052895604876, 80.55501292737007191 ) ) ;
#7447=PLANE ( 'NONE',  #24568 ) ;
#7450=EDGE_CURVE ( 'NONE', #7462, #7938, #20840, .T. ) ;
#7459=CARTESIAN_POINT ( 'NONE',  ( 40.64099152588523367, -8.607181138186998481, 78.30501292736998664 ) ) ;
#7461=PRESENTATION_STYLE_ASSIGNMENT (( #11725 ) ) ;
#7462=VERTEX_POINT ( 'NONE', #22763 ) ;
#7469=LINE ( 'NONE', #3592, #6967 ) ;
#7485=ORIENTED_EDGE ( 'NONE', *, *, #21470, .T. ) ;
#7492=CARTESIAN_POINT ( 'NONE',  ( 30.81606138205700418, -30.95005513552129983, 81.04249030099066431 ) ) ;
#7496=FACE_OUTER_BOUND ( 'NONE', #5774, .T. ) ;
#7500=DIRECTION ( 'NONE',  ( 0.000000000000000000, 1.000000000000000000, 0.000000000000000000 ) ) ;
#7515=EDGE_CURVE ( 'NONE', #22306, #24213, #18775, .T. ) ;
#7517=VECTOR ( 'NONE', #7728, 1000.000000000000000 ) ;
#7519=EDGE_LOOP ( 'NONE', ( #15686, #17082, #12946, #24007 ) ) ;
#7523=CARTESIAN_POINT ( 'NONE',  ( 35.64099152588522657, -1.357181138186998925, 80.05501292737000085 ) ) ;
#7524=FACE_OUTER_BOUND ( 'NONE', #20441, .T. ) ;
#7532=ADVANCED_FACE ( 'NONE', ( #24545 ), #6927, .F. ) ;
#7550=AXIS2_PLACEMENT_3D ( 'NONE', #17187, #15245, #25011 ) ;
#7552=PLANE ( 'NONE',  #11098 ) ;
#7558=AXIS2_PLACEMENT_3D ( 'NONE', #12011, #6450, #503 ) ;
#7567=ORIENTED_EDGE ( 'NONE', *, *, #10707, .T. ) ;
#7570=CARTESIAN_POINT ( 'NONE',  ( 44.81606138205700063, -30.95005513552129983, 81.04249030099066431 ) ) ;
#7598=CARTESIAN_POINT ( 'NONE',  ( 38.41621794735363693, -35.10729675983900222, 84.30501292737010033 ) ) ;
#7604=EDGE_CURVE ( 'NONE', #2759, #21678, #3443, .T. ) ;
#7609=AXIS2_PLACEMENT_3D ( 'NONE', #5059, #3240, #3117 ) ;
#7636=EDGE_LOOP ( 'NONE', ( #11742, #13818, #19811, #23056 ) ) ;
#7644=EDGE_CURVE ( 'NONE', #2290, #10641, #5379, .T. ) ;
#7648=VERTEX_POINT ( 'NONE', #9760 ) ;
#7652=LINE ( 'NONE', #19492, #12492 ) ;
#7657=DIRECTION ( 'NONE',  ( -1.000000000000000000, 0.000000000000000000, 2.507072128559814651E-16 ) ) ;
#7660=EDGE_CURVE ( 'NONE', #18894, #22752, #23015, .T. ) ;
#7667=LINE ( 'NONE', #25153, #4663 ) ;
#7668=LINE ( 'NONE', #23491, #11822 ) ;
#7673=DIRECTION ( 'NONE',  ( -1.734723475976804876E-16, -3.469446951953610245E-15, -1.000000000000000000 ) ) ;
#7679=DIRECTION ( 'NONE',  ( -1.734723475976809806E-16, 0.000000000000000000, -1.000000000000000000 ) ) ;
#7697=ADVANCED_FACE ( 'NONE', ( #4794 ), #6140, .F. ) ;
#7701=CARTESIAN_POINT ( 'NONE',  ( 32.56606138205700773, 40.39281886181299797, 82.55501292736983032 ) ) ;
#7708=CIRCLE ( 'NONE', #1910, 1.500000000000001332 ) ;
#7725=VECTOR ( 'NONE', #2575, 1000.000000000000000 ) ;
#7727=DIRECTION ( 'NONE',  ( 1.000000000000000000, 1.734723475976804876E-16, -1.734723475976814737E-16 ) ) ;
#7728=DIRECTION ( 'NONE',  ( 1.734723475976804876E-16, 3.491481338843135327E-15, 1.000000000000000000 ) ) ;
#7729=DIRECTION ( 'NONE',  ( 0.000000000000000000, -1.000000000000000000, 3.469446951953617344E-15 ) ) ;
#7731=CARTESIAN_POINT ( 'NONE',  ( 44.81606138205700063, -38.55876147765410167, 72.21586839016146087 ) ) ;
#7734=ORIENTED_EDGE ( 'NONE', *, *, #711, .F. ) ;
#7760=CARTESIAN_POINT ( 'NONE',  ( 45.81606138205700063, -34.55876147765410167, 70.30501292737000085 ) ) ;
#7778=ORIENTED_EDGE ( 'NONE', *, *, #15862, .F. ) ;
#7783=VERTEX_POINT ( 'NONE', #13870 ) ;
#7784=ORIENTED_EDGE ( 'NONE', *, *, #2685, .T. ) ;
#7791=DIRECTION ( 'NONE',  ( -1.000000000000000000, -1.734723475976804876E-16, 1.734723475976814737E-16 ) ) ;
#7795=CYLINDRICAL_SURFACE ( 'NONE', #10029, 3.999999999999899636 ) ;
#7810=ORIENTED_EDGE ( 'NONE', *, *, #21240, .F. ) ;
#7817=DIRECTION ( 'NONE',  ( -1.734723475976804876E-16, -3.491481338843135327E-15, -1.000000000000000000 ) ) ;
#7826=VECTOR ( 'NONE', #8989, 1000.000000000000000 ) ;
#7835=FACE_OUTER_BOUND ( 'NONE', #21199, .T. ) ;
#7836=DIRECTION ( 'NONE',  ( 0.000000000000000000, 1.000000000000000000, -3.304235192336775512E-15 ) ) ;
#7842=ORIENTED_EDGE ( 'NONE', *, *, #18269, .F. ) ;
#7853=ORIENTED_EDGE ( 'NONE', *, *, #13826, .F. ) ;
#7855=PLANE ( 'NONE',  #2204 ) ;
#7866=VECTOR ( 'NONE', #17219, 1000.000000000000000 ) ;
#7881=CARTESIAN_POINT ( 'NONE',  ( 45.81606138205700063, -26.74044063519535186, 84.30501292737007191 ) ) ;
#7884=DIRECTION ( 'NONE',  ( 0.000000000000000000, 1.000000000000000000, 0.000000000000000000 ) ) ;
#7887=CARTESIAN_POINT ( 'NONE',  ( 32.56606138205700773, 40.39281886181299797, 84.30501292736984453 ) ) ;
#7922=ORIENTED_EDGE ( 'NONE', *, *, #711, .T. ) ;
#7923=ADVANCED_FACE ( 'NONE', ( #7496 ), #23321, .F. ) ;
#7935=ORIENTED_EDGE ( 'NONE', *, *, #5779, .T. ) ;
#7938=VERTEX_POINT ( 'NONE', #25248 ) ;
#7939=EDGE_CURVE ( 'NONE', #7305, #16039, #24667, .T. ) ;
#7987=ADVANCED_FACE ( 'NONE', ( #136 ), #11885, .T. ) ;
#7994=CIRCLE ( 'NONE', #8416, 2.000000000000001776 ) ;
#7998=ORIENTED_EDGE ( 'NONE', *, *, #22449, .F. ) ;
#8008=ORIENTED_EDGE ( 'NONE', *, *, #6282, .T. ) ;
#8013=DIRECTION ( 'NONE',  ( 1.000000000000000000, 1.950367120401949903E-17, -2.478176394252580155E-16 ) ) ;
#8030=AXIS2_PLACEMENT_3D ( 'NONE', #12922, #18710, #11112 ) ;
#8036=LINE ( 'NONE', #17695, #10699 ) ;
#8047=CARTESIAN_POINT ( 'NONE',  ( 44.06606138205700063, 40.39281886181299797, 82.55501292736983032 ) ) ;
#8048=AXIS2_PLACEMENT_3D ( 'NONE', #133, #8013, #5683 ) ;
#8056=FACE_OUTER_BOUND ( 'NONE', #5739, .T. ) ;
#8068=EDGE_CURVE ( 'NONE', #17340, #10765, #2314, .T. ) ;
#8070=ORIENTED_EDGE ( 'NONE', *, *, #13175, .T. ) ;
#8076=DIRECTION ( 'NONE',  ( 1.734723475976804876E-16, 3.269436733918100469E-15, 1.000000000000000000 ) ) ;
#8098=EDGE_LOOP ( 'NONE', ( #10774, #22472, #6191, #15716 ) ) ;
#8099=FACE_OUTER_BOUND ( 'NONE', #24777, .T. ) ;
#8117=LINE ( 'NONE', #23815, #7011 ) ;
#8118=ORIENTED_EDGE ( 'NONE', *, *, #6807, .F. ) ;
#8131=CARTESIAN_POINT ( 'NONE',  ( 31.81606138205700418, 40.39281886181299797, 82.55501292736983032 ) ) ;
#8136=DIRECTION ( 'NONE',  ( -1.734723475976804876E-16, -3.469446951953620105E-15, -1.000000000000000000 ) ) ;
#8138=AXIS2_PLACEMENT_3D ( 'NONE', #24318, #8509, #22409 ) ;
#8140=CARTESIAN_POINT ( 'NONE',  ( 40.64099152588522657, -0.6071811381869983704, 82.55501292736998664 ) ) ;
#8153=ORIENTED_EDGE ( 'NONE', *, *, #2008, .T. ) ;
#8155=EDGE_CURVE ( 'NONE', #16594, #7151, #25481, .T. ) ;
#8160=EDGE_LOOP ( 'NONE', ( #23217, #22905, #15243, #4859 ) ) ;
#8176=CARTESIAN_POINT ( 'NONE',  ( 45.81606138205700063, -34.67340937580780036, 71.26505871168839690 ) ) ;
#8179=CARTESIAN_POINT ( 'NONE',  ( 32.56606138205700773, 40.39281886181299797, 82.55501292736983032 ) ) ;
#8187=ORIENTED_EDGE ( 'NONE', *, *, #3529, .F. ) ;
#8198=DIRECTION ( 'NONE',  ( 6.505213034913089466E-17, -1.000000000000000000, 3.491481338843135327E-15 ) ) ;
#8206=AXIS2_PLACEMENT_3D ( 'NONE', #2960, #4907, #10586 ) ;
#8209=LINE ( 'NONE', #12210, #735 ) ;
#8214=CIRCLE ( 'NONE', #14387, 12.59999999999999964 ) ;
#8216=LINE ( 'NONE', #18141, #5272 ) ;
#8219=DIRECTION ( 'NONE',  ( 0.000000000000000000, -3.491481338843135327E-15, -1.000000000000000000 ) ) ;
#8238=ADVANCED_FACE ( 'NONE', ( #8261 ), #2442, .F. ) ;
#8258=DIRECTION ( 'NONE',  ( -1.734723475976814737E-16, 0.000000000000000000, -1.000000000000000000 ) ) ;
#8261=FACE_OUTER_BOUND ( 'NONE', #7636, .T. ) ;
#8282=ORIENTED_EDGE ( 'NONE', *, *, #5603, .T. ) ;
#8288=ORIENTED_EDGE ( 'NONE', *, *, #1251, .F. ) ;
#8290=LINE ( 'NONE', #6478, #2238 ) ;
#8291=LINE ( 'NONE', #12292, #12497 ) ;
#8293=CARTESIAN_POINT ( 'NONE',  ( 40.64099152588522657, 1.832818861813001021, 78.30501292736998664 ) ) ;
#8296=DIRECTION ( 'NONE',  ( 1.000000000000000000, 1.734723475976814737E-16, -1.734723475976804876E-16 ) ) ;
#8306=EDGE_CURVE ( 'NONE', #17348, #6502, #22916, .T. ) ;
#8313=ORIENTED_EDGE ( 'NONE', *, *, #18260, .T. ) ;
#8327=VECTOR ( 'NONE', #3815, 1000.000000000000000 ) ;
#8329=AXIS2_PLACEMENT_3D ( 'NONE', #8357, #16447, #10793 ) ;
#8346=DIRECTION ( 'NONE',  ( 0.000000000000000000, 0.000000000000000000, 1.000000000000000000 ) ) ;
#8351=ORIENTED_EDGE ( 'NONE', *, *, #9974, .F. ) ;
#8357=CARTESIAN_POINT ( 'NONE',  ( 32.56606138205700773, 41.41058581477939526, 84.01211970855638356 ) ) ;
#8359=AXIS2_PLACEMENT_3D ( 'NONE', #8612, #8743, #12859 ) ;
#8382=AXIS2_PLACEMENT_3D ( 'NONE', #10448, #15971, #24079 ) ;
#8389=ORIENTED_EDGE ( 'NONE', *, *, #18706, .F. ) ;
#8390=AXIS2_PLACEMENT_3D ( 'NONE', #17083, #9236, #21069 ) ;
#8394=DIRECTION ( 'NONE',  ( 1.000000000000000000, 0.000000000000000000, 0.000000000000000000 ) ) ;
#8395=PLANE ( 'NONE',  #17766 ) ;
#8416=AXIS2_PLACEMENT_3D ( 'NONE', #4681, #12557, #437 ) ;
#8423=CARTESIAN_POINT ( 'NONE',  ( 30.81606138205700418, -34.67340937580780036, 71.26505871168839690 ) ) ;
#8427=CYLINDRICAL_SURFACE ( 'NONE', #1539, 0.7500000000000022204 ) ;
#8448=EDGE_CURVE ( 'NONE', #12300, #25398, #11347, .T. ) ;
#8455=CARTESIAN_POINT ( 'NONE',  ( 31.81606138205700418, -34.55876147765410167, 70.30501292737000085 ) ) ;
#8461=VERTEX_POINT ( 'NONE', #13778 ) ;
#8465=EDGE_CURVE ( 'NONE', #22735, #18487, #1989, .T. ) ;
#8471=DIRECTION ( 'NONE',  ( 0.000000000000000000, -1.000000000000000000, 0.000000000000000000 ) ) ;
#8498=ORIENTED_EDGE ( 'NONE', *, *, #5667, .T. ) ;
#8503=ORIENTED_EDGE ( 'NONE', *, *, #12427, .F. ) ;
#8509=DIRECTION ( 'NONE',  ( -1.734723475976804876E-16, -3.469446951953610245E-15, -1.000000000000000000 ) ) ;
#8534=CIRCLE ( 'NONE', #11427, 1.000000000000000888 ) ;
#8548=CARTESIAN_POINT ( 'NONE',  ( 44.81606138205700063, -26.74044063519535186, 82.55501292737007191 ) ) ;
#8552=VECTOR ( 'NONE', #1668, 1000.000000000000000 ) ;
#8553=ORIENTED_EDGE ( 'NONE', *, *, #15862, .T. ) ;
#8557=LINE ( 'NONE', #6612, #21268 ) ;
#8564=DIRECTION ( 'NONE',  ( -1.734723475976814737E-16, 1.000000000000000000, -3.491481338843135327E-15 ) ) ;
#8569=ORIENTED_EDGE ( 'NONE', *, *, #4604, .T. ) ;
#8580=LINE ( 'NONE', #24263, #2889 ) ;
#8612=CARTESIAN_POINT ( 'NONE',  ( 35.64099152588522657, -1.357181138186998925, 80.05501292737000085 ) ) ;
#8638=DIRECTION ( 'NONE',  ( 0.000000000000000000, -0.7071067811865489050, 0.7071067811865460184 ) ) ;
#8643=EDGE_LOOP ( 'NONE', ( #1276, #21965, #6942, #841 ) ) ;
#8668=EDGE_CURVE ( 'NONE', #7351, #5806, #2791, .T. ) ;
#8691=CARTESIAN_POINT ( 'NONE',  ( 31.81606138205700418, 40.39281886181299797, 66.30501292737000085 ) ) ;
#8695=VECTOR ( 'NONE', #9119, 1000.000000000000000 ) ;
#8703=CARTESIAN_POINT ( 'NONE',  ( 32.56606138205700773, 45.04446929126255128, 81.37823623207320622 ) ) ;
#8730=LINE ( 'NONE', #20439, #23071 ) ;
#8732=ORIENTED_EDGE ( 'NONE', *, *, #4379, .T. ) ;
#8743=DIRECTION ( 'NONE',  ( 1.000000000000000000, 0.000000000000000000, 0.000000000000000000 ) ) ;
#8747=CARTESIAN_POINT ( 'NONE',  ( 45.81606138205700063, -34.55876147765410167, 70.30501292737000085 ) ) ;
#8754=ORIENTED_EDGE ( 'NONE', *, *, #18269, .T. ) ;
#8756=VECTOR ( 'NONE', #18403, 1000.000000000000000 ) ;
#8759=VECTOR ( 'NONE', #3178, 1000.000000000000000 ) ;
#8764=DIRECTION ( 'NONE',  ( 0.000000000000000000, -3.491481338843135327E-15, -1.000000000000000000 ) ) ;
#8770=LINE ( 'NONE', #2814, #9292 ) ;
#8783=ADVANCED_FACE ( 'NONE', ( #10867 ), #18719, .T. ) ;
#8784=AXIS2_PLACEMENT_3D ( 'NONE', #6760, #4818, #14613 ) ;
#8791=AXIS2_PLACEMENT_3D ( 'NONE', #4, #4009, #7884 ) ;
#8803=ADVANCED_FACE ( 'NONE', ( #16914, #18973 ), #1178, .T. ) ;
#8805=CARTESIAN_POINT ( 'NONE',  ( 40.64099152588522657, 0.3928188618129990761, 82.55501292736997243 ) ) ;
#8806=CARTESIAN_POINT ( 'NONE',  ( 42.06606138205700063, 47.04446929126260102, 81.37823623207319201 ) ) ;
#8810=EDGE_CURVE ( 'NONE', #17608, #11322, #22954, .T. ) ;
#8814=DIRECTION ( 'NONE',  ( 0.000000000000000000, 1.000000000000000000, 0.000000000000000000 ) ) ;
#8816=DIRECTION ( 'NONE',  ( -1.734723475976739795E-16, -4.343580702399009298E-14, -1.000000000000000000 ) ) ;
#8818=CARTESIAN_POINT ( 'NONE',  ( 44.06606138205700063, 40.39281886181299797, 82.55501292736983032 ) ) ;
#8829=EDGE_CURVE ( 'NONE', #14211, #7351, #6377, .T. ) ;
#8832=ORIENTED_EDGE ( 'NONE', *, *, #9974, .T. ) ;
#8841=LINE ( 'NONE', #5216, #4247 ) ;
#8862=PLANE ( 'NONE',  #21856 ) ;
#8863=VERTEX_POINT ( 'NONE', #24992 ) ;
#8871=DIRECTION ( 'NONE',  ( -1.000000000000000000, 0.000000000000000000, 0.000000000000000000 ) ) ;
#8880=VECTOR ( 'NONE', #9405, 1000.000000000000000 ) ;
#8881=DIRECTION ( 'NONE',  ( 1.734723475976804876E-16, 3.552713678800500140E-15, 1.000000000000000000 ) ) ;
#8883=DIRECTION ( 'NONE',  ( -1.000000000000000000, -1.734723475976804876E-16, 1.734723475976814737E-16 ) ) ;
#8885=EDGE_CURVE ( 'NONE', #2290, #7039, #3165, .T. ) ;
#8915=CARTESIAN_POINT ( 'NONE',  ( 44.06606138205700063, 40.39281886181299797, 82.55501292736983032 ) ) ;
#8920=FACE_OUTER_BOUND ( 'NONE', #11179, .T. ) ;
#8937=CARTESIAN_POINT ( 'NONE',  ( 44.81606138205700063, -26.74044063519535186, 82.50501292737007475 ) ) ;
#8955=ORIENTED_EDGE ( 'NONE', *, *, #4067, .T. ) ;
#8961=DIRECTION ( 'NONE',  ( 1.000000000000000000, 1.734723475976804876E-16, -1.734723475976814737E-16 ) ) ;
#8963=VECTOR ( 'NONE', #11754, 1000.000000000000000 ) ;
#8975=CYLINDRICAL_SURFACE ( 'NONE', #20077, 4.000000000000003553 ) ;
#8976=LINE ( 'NONE', #1353, #14511 ) ;
#8988=LINE ( 'NONE', #11176, #21072 ) ;
#8989=DIRECTION ( 'NONE',  ( -1.734723475976804876E-16, 1.000000000000000000, 3.009265538105065326E-32 ) ) ;
#8991=ORIENTED_EDGE ( 'NONE', *, *, #24059, .T. ) ;
#9004=DIRECTION ( 'NONE',  ( 0.000000000000000000, -4.343580702399009298E-14, -1.000000000000000000 ) ) ;
#9005=VECTOR ( 'NONE', #11855, 1000.000000000000000 ) ;
#9014=ORIENTED_EDGE ( 'NONE', *, *, #1300, .F. ) ;
#9042=DIRECTION ( 'NONE',  ( 1.734723475976804876E-16, 3.469446951953610245E-15, 1.000000000000000000 ) ) ;
#9066=VECTOR ( 'NONE', #24672, 1000.000000000000000 ) ;
#9074=DIRECTION ( 'NONE',  ( 0.000000000000000000, -1.000000000000000000, 3.469446951953611033E-15 ) ) ;
#9081=EDGE_CURVE ( 'NONE', #11508, #20175, #15976, .T. ) ;
#9100=EDGE_CURVE ( 'NONE', #194, #18550, #20366, .T. ) ;
#9116=CARTESIAN_POINT ( 'NONE',  ( 40.64099152588522657, 1.142818861812999742, 83.30501292736997243 ) ) ;
#9117=FACE_BOUND ( 'NONE', #14245, .T. ) ;
#9119=DIRECTION ( 'NONE',  ( -6.505213034913089466E-17, 1.000000000000000000, -3.491481338843135327E-15 ) ) ;
#9139=CYLINDRICAL_SURFACE ( 'NONE', #10801, 4.000000000000000000 ) ;
#9154=CARTESIAN_POINT ( 'NONE',  ( 41.14099152588523367, 1.392818861812999964, 93.30501292736998664 ) ) ;
#9161=VECTOR ( 'NONE', #8881, 1000.000000000000000 ) ;
#9225=VECTOR ( 'NONE', #789, 1000.000000000000114 ) ;
#9227=ORIENTED_EDGE ( 'NONE', *, *, #6149, .T. ) ;
#9231=AXIS2_PLACEMENT_3D ( 'NONE', #15702, #19696, #9074 ) ;
#9233=LINE ( 'NONE', #22609, #9770 ) ;
#9235=ORIENTED_EDGE ( 'NONE', *, *, #19582, .T. ) ;
#9236=DIRECTION ( 'NONE',  ( 1.000000000000000000, 2.168404344971005170E-16, -1.734723475976814737E-16 ) ) ;
#9254=DIRECTION ( 'NONE',  ( 1.000000000000000000, 0.000000000000000000, 0.000000000000000000 ) ) ;
#9258=VERTEX_POINT ( 'NONE', #20110 ) ;
#9262=CARTESIAN_POINT ( 'NONE',  ( 35.14099152588523367, 1.392818861812999964, 93.30501292736998664 ) ) ;
#9271=DIRECTION ( 'NONE',  ( -1.000000000000000000, 0.000000000000000000, 2.507072128559814651E-16 ) ) ;
#9276=ADVANCED_FACE ( 'NONE', ( #3343 ), #1021, .T. ) ;
#9286=CARTESIAN_POINT ( 'NONE',  ( 0.000000000000000000, 0.000000000000000000, 0.000000000000000000 ) ) ;
#9290=EDGE_CURVE ( 'NONE', #10220, #2117, #11088, .T. ) ;
#9292=VECTOR ( 'NONE', #16607, 1000.000000000000000 ) ;
#9294=VERTEX_POINT ( 'NONE', #18944 ) ;
#9313=ORIENTED_EDGE ( 'NONE', *, *, #24590, .F. ) ;
#9325=CARTESIAN_POINT ( 'NONE',  ( 32.56606138205700773, 42.82479937715250173, 82.59790614618329130 ) ) ;
#9340=PLANE ( 'NONE',  #10697 ) ;
#9362=VERTEX_POINT ( 'NONE', #7343 ) ;
#9363=DIRECTION ( 'NONE',  ( 0.000000000000000000, -1.000000000000000000, 3.491481338843135327E-15 ) ) ;
#9364=FACE_OUTER_BOUND ( 'NONE', #360, .T. ) ;
#9384=CARTESIAN_POINT ( 'NONE',  ( 40.64099152588522657, 1.142818861812999742, 82.55501292736997243 ) ) ;
#9403=AXIS2_PLACEMENT_3D ( 'NONE', #19166, #17117, #1502 ) ;
#9405=DIRECTION ( 'NONE',  ( 1.000000000000000000, 1.734723475976804876E-16, -1.734723475976814737E-16 ) ) ;
#9411=CARTESIAN_POINT ( 'NONE',  ( 35.64099152588522657, 1.392818861812999964, 83.30501292736997243 ) ) ;
#9414=EDGE_CURVE ( 'NONE', #18550, #3634, #11647, .T. ) ;
#9425=EDGE_CURVE ( 'NONE', #13947, #17020, #1327, .T. ) ;
#9428=EDGE_CURVE ( 'NONE', #13296, #4487, #23428, .T. ) ;
#9437=CARTESIAN_POINT ( 'NONE',  ( 44.81606138205700063, -34.55876147765410167, 66.30501292737000085 ) ) ;
#9443=CIRCLE ( 'NONE', #8206, 0.7500000000000006661 ) ;
#9451=DIRECTION ( 'NONE',  ( 1.000000000000000000, 3.197344634236645231E-31, -1.734723475976814737E-16 ) ) ;
#9469=ORIENTED_EDGE ( 'NONE', *, *, #4050, .F. ) ;
#9473=FACE_OUTER_BOUND ( 'NONE', #13668, .T. ) ;
#9490=DIRECTION ( 'NONE',  ( 1.734723475976804876E-16, 3.491481338843135327E-15, 1.000000000000000000 ) ) ;
#9494=AXIS2_PLACEMENT_3D ( 'NONE', #22036, #16352, #6572 ) ;
#9499=EDGE_CURVE ( 'NONE', #5274, #24509, #13649, .T. ) ;
#9505=ORIENTED_EDGE ( 'NONE', *, *, #24961, .F. ) ;
#9508=CARTESIAN_POINT ( 'NONE',  ( 45.81606138205700063, -38.55876147765410167, 70.30501292737011454 ) ) ;
#9527=ORIENTED_EDGE ( 'NONE', *, *, #4516, .T. ) ;
#9528=ORIENTED_EDGE ( 'NONE', *, *, #9100, .F. ) ;
#9533=ORIENTED_EDGE ( 'NONE', *, *, #14095, .F. ) ;
#9543=CARTESIAN_POINT ( 'NONE',  ( 40.64099152588522657, -0.6071811381869983704, 122.0250129273699997 ) ) ;
#9549=ORIENTED_EDGE ( 'NONE', *, *, #22314, .F. ) ;
#9592=ORIENTED_EDGE ( 'NONE', *, *, #243, .F. ) ;
#9593=DIRECTION ( 'NONE',  ( -1.000000000000000000, 4.930380657631319405E-32, 1.734723475976804876E-16 ) ) ;
#9595=CARTESIAN_POINT ( 'NONE',  ( 35.64099152588522657, -1.357181138186998925, 78.30501292736998664 ) ) ;
#9602=LINE ( 'NONE', #17572, #24369 ) ;
#9611=ORIENTED_EDGE ( 'NONE', *, *, #17938, .T. ) ;
#9617=EDGE_LOOP ( 'NONE', ( #15515, #13890, #18817, #23916 ) ) ;
#9627=ORIENTED_EDGE ( 'NONE', *, *, #22310, .T. ) ;
#9650=EDGE_CURVE ( 'NONE', #18487, #22083, #24173, .T. ) ;
#9655=ORIENTED_EDGE ( 'NONE', *, *, #11770, .T. ) ;
#9658=ORIENTED_EDGE ( 'NONE', *, *, #10566, .T. ) ;
#9666=ORIENTED_EDGE ( 'NONE', *, *, #3273, .T. ) ;
#9674=AXIS2_PLACEMENT_3D ( 'NONE', #11881, #21153, #5945 ) ;
#9675=EDGE_CURVE ( 'NONE', #7151, #23326, #10552, .T. ) ;
#9683=DIRECTION ( 'NONE',  ( 1.000000000000000000, -6.018531076210131309E-31, -1.734723475976804876E-16 ) ) ;
#9721=DIRECTION ( 'NONE',  ( -2.290324355028189071E-16, 0.4067366430757970996, -0.9135454576426023099 ) ) ;
#9725=CARTESIAN_POINT ( 'NONE',  ( 31.81606138205700418, -38.55876147765410167, 70.30501292737011454 ) ) ;
#9736=DIRECTION ( 'NONE',  ( -1.734723475976804876E-16, -3.491481338843135327E-15, -1.000000000000000000 ) ) ;
#9739=ORIENTED_EDGE ( 'NONE', *, *, #2246, .T. ) ;
#9742=LINE ( 'NONE', #17091, #13457 ) ;
#9760=CARTESIAN_POINT ( 'NONE',  ( 40.64099152588523367, -8.607181138186998481, 78.30501292736998664 ) ) ;
#9770=VECTOR ( 'NONE', #7279, 1000.000000000000000 ) ;
#9780=CARTESIAN_POINT ( 'NONE',  ( 40.64099152588522657, 40.39281886181299797, 84.30501292736984453 ) ) ;
#9783=DIRECTION ( 'NONE',  ( 0.000000000000000000, 1.000000000000000000, -6.938893903907222067E-15 ) ) ;
#9792=CIRCLE ( 'NONE', #13886, 4.000000000000000000 ) ;
#9803=AXIS2_PLACEMENT_3D ( 'NONE', #753, #6822, #18797 ) ;
#9823=DIRECTION ( 'NONE',  ( -9.121204216617950752E-31, -0.7071067811865461294, -0.7071067811865490160 ) ) ;
#9842=ORIENTED_EDGE ( 'NONE', *, *, #8155, .F. ) ;
#9844=DIRECTION ( 'NONE',  ( -1.000000000000000000, 0.000000000000000000, 1.586291242107190025E-15 ) ) ;
#9859=DIRECTION ( 'NONE',  ( -7.966588320977881105E-33, 1.000000000000000000, -6.123233995736769734E-17 ) ) ;
#9863=DIRECTION ( 'NONE',  ( 1.000000000000000000, 0.000000000000000000, -1.301042606982603842E-16 ) ) ;
#9864=ORIENTED_EDGE ( 'NONE', *, *, #2787, .T. ) ;
#9883=EDGE_CURVE ( 'NONE', #18741, #12591, #23960, .T. ) ;
#9889=ORIENTED_EDGE ( 'NONE', *, *, #6269, .T. ) ;
#9896=LINE ( 'NONE', #80, #16780 ) ;
#9898=CIRCLE ( 'NONE', #25061, 0.7500000000000006661 ) ;
#9913=ADVANCED_FACE ( 'NONE', ( #24814 ), #4870, .F. ) ;
#9914=EDGE_LOOP ( 'NONE', ( #25093, #12129, #4989, #22476 ) ) ;
#9918=DIRECTION ( 'NONE',  ( -1.000000000000000000, -2.168404344971055214E-16, 1.734723475976814737E-16 ) ) ;
#9922=AXIS2_PLACEMENT_3D ( 'NONE', #9154, #11076, #8764 ) ;
#9928=ORIENTED_EDGE ( 'NONE', *, *, #2008, .F. ) ;
#9932=ORIENTED_EDGE ( 'NONE', *, *, #4082, .F. ) ;
#9935=PRODUCT ( 'Metal Base Plate', 'Metal Base Plate', '', ( #11261 ) ) ;
#9965=VERTEX_POINT ( 'NONE', #5760 ) ;
#9972=EDGE_LOOP ( 'NONE', ( #9666, #11702, #13588, #18735, #10479, #4948, #16012, #5759, #1482, #21496, #11948, #25056, #7784, #6003, #3281, #161 ) ) ;
#9973=CARTESIAN_POINT ( 'NONE',  ( 30.81606138205700418, 1.392818861812999964, 84.30501292737000085 ) ) ;
#9974=EDGE_CURVE ( 'NONE', #13207, #6422, #6701, .T. ) ;
#9982=ORIENTED_EDGE ( 'NONE', *, *, #6812, .T. ) ;
#9992=ORIENTED_EDGE ( 'NONE', *, *, #21858, .F. ) ;
#10002=ORIENTED_EDGE ( 'NONE', *, *, #21536, .F. ) ;
#10006=AXIS2_PLACEMENT_3D ( 'NONE', #4554, #2347, #408 ) ;
#10020=DIRECTION ( 'NONE',  ( 0.000000000000000000, 1.000000000000000000, -3.469446951953614189E-15 ) ) ;
#10021=VECTOR ( 'NONE', #9859, 1000.000000000000000 ) ;
#10025=CIRCLE ( 'NONE', #8791, 0.7500000000000006661 ) ;
#10029=AXIS2_PLACEMENT_3D ( 'NONE', #25287, #13462, #17585 ) ;
#10037=VECTOR ( 'NONE', #3157, 1000.000000000000000 ) ;
#10039=CARTESIAN_POINT ( 'NONE',  ( 44.06606138205700063, 40.39281886181299797, 84.30501292736984453 ) ) ;
#10045=EDGE_CURVE ( 'NONE', #22094, #21036, #17496, .T. ) ;
#10101=ORIENTED_EDGE ( 'NONE', *, *, #10045, .T. ) ;
#10129=ORIENTED_EDGE ( 'NONE', *, *, #6807, .T. ) ;
#10133=LINE ( 'NONE', #17994, #13637 ) ;
#10140=VERTEX_POINT ( 'NONE', #17880 ) ;
#10177=ORIENTED_EDGE ( 'NONE', *, *, #10516, .F. ) ;
#10195=FACE_OUTER_BOUND ( 'NONE', #13856, .T. ) ;
#10202=AXIS2_PLACEMENT_3D ( 'NONE', #4392, #18176, #19847 ) ;
#10217=DIRECTION ( 'NONE',  ( 0.000000000000000000, 0.000000000000000000, 1.000000000000000000 ) ) ;
#10220=VERTEX_POINT ( 'NONE', #2390 ) ;
#10235=PLANE ( 'NONE',  #25188 ) ;
#10243=VECTOR ( 'NONE', #1565, 999.9999999999998863 ) ;
#10255=DIRECTION ( 'NONE',  ( -1.000000000000000000, -2.168404344971005170E-16, 1.734723475976814737E-16 ) ) ;
#10262=EDGE_LOOP ( 'NONE', ( #24729, #688, #15533, #21804 ) ) ;
#10276=CARTESIAN_POINT ( 'NONE',  ( 40.64099152588522657, -9.607181138187000258, 83.02501292736999972 ) ) ;
#10287=DIRECTION ( 'NONE',  ( -1.000000000000000000, 6.018531076210110289E-31, 1.734723475976804876E-16 ) ) ;
#10289=AXIS2_PLACEMENT_3D ( 'NONE', #22595, #4950, #12820 ) ;
#10291=ADVANCED_FACE ( 'NONE', ( #2760 ), #14756, .T. ) ;
#10296=CARTESIAN_POINT ( 'NONE',  ( 32.56606138205700773, 40.39281886181299797, 82.55501292736983032 ) ) ;
#10300=CARTESIAN_POINT ( 'NONE',  ( 30.81606138205700418, -36.30035594811090505, 74.91924054225879104 ) ) ;
#10303=AXIS2_PLACEMENT_3D ( 'NONE', #2463, #275, #10340 ) ;
#10319=CARTESIAN_POINT ( 'NONE',  ( 30.81606138205700418, -0.6071811381869983704, 122.0250129273699997 ) ) ;
#10331=ADVANCED_FACE ( 'NONE', ( #22362 ), #10901, .F. ) ;
#10332=DIRECTION ( 'NONE',  ( -1.000000000000000000, -1.734723475976804876E-16, 1.734723475976814737E-16 ) ) ;
#10340=DIRECTION ( 'NONE',  ( 0.000000000000000000, -1.000000000000000000, 2.775557561562890957E-15 ) ) ;
#10341=DIRECTION ( 'NONE',  ( 1.000000000000000000, -6.018531076210130433E-31, -1.734723475976804876E-16 ) ) ;
#10351=CARTESIAN_POINT ( 'NONE',  ( 32.56606138205700773, 29.91058581477919986, 95.51211970855651145 ) ) ;
#10352=ORIENTED_EDGE ( 'NONE', *, *, #491, .T. ) ;
#10354=CARTESIAN_POINT ( 'NONE',  ( 40.64099152588522657, -0.6071811381869983704, 80.05501292737000085 ) ) ;
#10366=ADVANCED_FACE ( 'NONE', ( #2644 ), #6779, .F. ) ;
#10367=CARTESIAN_POINT ( 'NONE',  ( 42.06606138205700063, 47.04446929126260102, 81.37823623207319201 ) ) ;
#10371=VERTEX_POINT ( 'NONE', #18373 ) ;
#10378=DIRECTION ( 'NONE',  ( -1.000000000000000000, -1.734723475976804876E-16, 1.734723475976814737E-16 ) ) ;
#10380=ORIENTED_EDGE ( 'NONE', *, *, #24319, .T. ) ;
#10395=EDGE_CURVE ( 'NONE', #12560, #17608, #18880, .T. ) ;
#10402=CARTESIAN_POINT ( 'NONE',  ( 32.56606138205700773, -26.74044063519535186, 84.30501292737007191 ) ) ;
#10405=CARTESIAN_POINT ( 'NONE',  ( 30.81606138205700418, 40.83281886181300280, 79.30501292736983032 ) ) ;
#10406=ORIENTED_EDGE ( 'NONE', *, *, #15936, .T. ) ;
#10417=DIRECTION ( 'NONE',  ( 1.000000000000000000, 1.734723475976804876E-16, -1.734723475976814737E-16 ) ) ;
#10418=AXIS2_PLACEMENT_3D ( 'NONE', #4299, #4166, #10217 ) ;
#10445=EDGE_LOOP ( 'NONE', ( #9528, #19486, #5620, #20818 ) ) ;
#10446=AXIS2_PLACEMENT_3D ( 'NONE', #3656, #1849, #5476 ) ;
#10447=FACE_BOUND ( 'NONE', #15819, .T. ) ;
#10448=CARTESIAN_POINT ( 'NONE',  ( 31.81606138205700418, 40.39281886181299797, 80.75501292736983316 ) ) ;
#10453=ADVANCED_FACE ( 'NONE', ( #25411 ), #22866, .F. ) ;
#10456=CARTESIAN_POINT ( 'NONE',  ( 35.64099152588522657, -9.607181138187000258, 82.55501292736998664 ) ) ;
#10466=ADVANCED_FACE ( 'NONE', ( #5601 ), #7795, .T. ) ;
#10470=CARTESIAN_POINT ( 'NONE',  ( 45.81606138205700063, 40.39281886181299797, 84.30501292736984453 ) ) ;
#10475=ORIENTED_EDGE ( 'NONE', *, *, #11356, .F. ) ;
#10479=ORIENTED_EDGE ( 'NONE', *, *, #584, .T. ) ;
#10482=VECTOR ( 'NONE', #21688, 1000.000000000000000 ) ;
#10501=VERTEX_POINT ( 'NONE', #13220 ) ;
#10503=ORIENTED_EDGE ( 'NONE', *, *, #6269, .F. ) ;
#10516=EDGE_CURVE ( 'NONE', #2496, #19007, #5503, .T. ) ;
#10518=ADVANCED_FACE ( 'NONE', ( #21314 ), #23239, .T. ) ;
#10521=ORIENTED_EDGE ( 'NONE', *, *, #23865, .T. ) ;
#10522=ORIENTED_EDGE ( 'NONE', *, *, #13344, .F. ) ;
#10524=EDGE_CURVE ( 'NONE', #11291, #120, #3414, .T. ) ;
#10529=DIRECTION ( 'NONE',  ( -1.301042606982603842E-16, 0.000000000000000000, -1.000000000000000000 ) ) ;
#10539=CARTESIAN_POINT ( 'NONE',  ( 45.81606138205700063, 0.1601050959395486362, 68.80395113470939350 ) ) ;
#10552=LINE ( 'NONE', #18287, #8756 ) ;
#10553=CARTESIAN_POINT ( 'NONE',  ( 32.56606138205700773, 43.35512946304240245, 82.37823623207322044 ) ) ;
#10566=EDGE_CURVE ( 'NONE', #6502, #24213, #7667, .T. ) ;
#10567=CARTESIAN_POINT ( 'NONE',  ( 38.31606138205700063, 29.20347903359266084, 94.80501292737000085 ) ) ;
#10585=ORIENTED_EDGE ( 'NONE', *, *, #23168, .F. ) ;
#10586=DIRECTION ( 'NONE',  ( 0.000000000000000000, 0.000000000000000000, 1.000000000000000000 ) ) ;
#10600=CYLINDRICAL_SURFACE ( 'NONE', #17269, 12.59999999999999964 ) ;
#10623=CARTESIAN_POINT ( 'NONE',  ( 38.41621794735363693, -35.10729675983900222, 83.30501292737010033 ) ) ;
#10625=CARTESIAN_POINT ( 'NONE',  ( 31.81606138205700418, 34.87886987267149408, 81.44836866983821722 ) ) ;
#10628=VERTEX_POINT ( 'NONE', #21949 ) ;
#10629=ORIENTED_EDGE ( 'NONE', *, *, #666, .T. ) ;
#10641=VERTEX_POINT ( 'NONE', #10354 ) ;
#10644=FILL_AREA_STYLE_COLOUR ( '', #17450 ) ;
#10651=CARTESIAN_POINT ( 'NONE',  ( 42.06606138205700063, 45.04446929126260102, 81.37823623207320622 ) ) ;
#10665=DIRECTION ( 'NONE',  ( -1.000000000000000000, 6.018531076210110289E-31, 1.734723475976804876E-16 ) ) ;
#10676=CARTESIAN_POINT ( 'NONE',  ( 41.14099152588522657, -10.60718113818700026, 83.30501292737001506 ) ) ;
#10677=ADVANCED_FACE ( 'NONE', ( #3925 ), #1972, .F. ) ;
#10697=AXIS2_PLACEMENT_3D ( 'NONE', #5337, #21053, #17186 ) ;
#10698=EDGE_CURVE ( 'NONE', #13966, #6270, #21821, .T. ) ;
#10699=VECTOR ( 'NONE', #3518, 1000.000000000000000 ) ;
#10704=ORIENTED_EDGE ( 'NONE', *, *, #17686, .F. ) ;
#10707=EDGE_CURVE ( 'NONE', #14027, #22094, #21551, .T. ) ;
#10721=ORIENTED_EDGE ( 'NONE', *, *, #6083, .F. ) ;
#10762=FACE_OUTER_BOUND ( 'NONE', #3191, .T. ) ;
#10765=VERTEX_POINT ( 'NONE', #2607 ) ;
#10766=ORIENTED_EDGE ( 'NONE', *, *, #16022, .F. ) ;
#10773=VERTEX_POINT ( 'NONE', #14471 ) ;
#10774=ORIENTED_EDGE ( 'NONE', *, *, #23168, .T. ) ;
#10775=ORIENTED_EDGE ( 'NONE', *, *, #2521, .F. ) ;
#10785=ORIENTED_EDGE ( 'NONE', *, *, #6950, .T. ) ;
#10790=ORIENTED_EDGE ( 'NONE', *, *, #8068, .F. ) ;
#10793=DIRECTION ( 'NONE',  ( -1.734723475976814737E-16, 0.000000000000000000, -1.000000000000000000 ) ) ;
#10798=DIRECTION ( 'NONE',  ( -1.734723475976804876E-16, -3.430248998885765387E-15, -1.000000000000000000 ) ) ;
#10801=AXIS2_PLACEMENT_3D ( 'NONE', #996, #10934, #1388 ) ;
#10809=VECTOR ( 'NONE', #22013, 1000.000000000000000 ) ;
#10811=CARTESIAN_POINT ( 'NONE',  ( 33.03722820848892638, 1.142818861812999742, 82.55501292736998664 ) ) ;
#10826=ORIENTED_EDGE ( 'NONE', *, *, #458, .F. ) ;
#10835=ADVANCED_FACE ( 'NONE', ( #800 ), #2987, .F. ) ;
#10836=ADVANCED_FACE ( 'NONE', ( #16391 ), #20786, .F. ) ;
#10839=AXIS2_PLACEMENT_3D ( 'NONE', #23222, #10341, #4549 ) ;
#10840=DIRECTION ( 'NONE',  ( -1.000000000000000000, 0.000000000000000000, 1.586291242107190025E-15 ) ) ;
#10843=CARTESIAN_POINT ( 'NONE',  ( 31.81606138205700418, -26.74044063519535186, 82.50501292737007475 ) ) ;
#10850=VECTOR ( 'NONE', #15772, 1000.000000000000000 ) ;
#10859=ORIENTED_EDGE ( 'NONE', *, *, #7939, .F. ) ;
#10867=FACE_OUTER_BOUND ( 'NONE', #3351, .T. ) ;
#10868=CIRCLE ( 'NONE', #15377, 1.750000000000001554 ) ;
#10871=DIRECTION ( 'NONE',  ( 0.000000000000000000, -3.491481338843135327E-15, -1.000000000000000000 ) ) ;
#10872=DIRECTION ( 'NONE',  ( 6.489379976170840313E-31, -1.000000000000000000, 3.491481338843135327E-15 ) ) ;
#10891=DIRECTION ( 'NONE',  ( -1.000000000000000000, 4.930380657631319405E-32, 1.734723475976804876E-16 ) ) ;
#10901=PLANE ( 'NONE',  #1760 ) ;
#10909=DIRECTION ( 'NONE',  ( -1.000000000000000000, -1.734723475976804876E-16, 1.734723475976814737E-16 ) ) ;
#10915=CIRCLE ( 'NONE', #16684, 0.7500000000000006661 ) ;
#10917=ADVANCED_FACE ( 'NONE', ( #24238 ), #6611, .T. ) ;
#10924=ORIENTED_EDGE ( 'NONE', *, *, #5117, .F. ) ;
#10931=ADVANCED_FACE ( 'NONE', ( #20910 ), #25347, .F. ) ;
#10934=DIRECTION ( 'NONE',  ( -1.000000000000000000, -2.168404344971005170E-16, 1.734723475976814737E-16 ) ) ;
#10939=LINE ( 'NONE', #16990, #16443 ) ;
#10940=DIRECTION ( 'NONE',  ( -1.734723475976804876E-16, -3.491481338843135327E-15, -1.000000000000000000 ) ) ;
#10941=ORIENTED_EDGE ( 'NONE', *, *, #1650, .F. ) ;
#10968=DIRECTION ( 'NONE',  ( -1.734723475976814737E-16, 0.000000000000000000, -1.000000000000000000 ) ) ;
#10979=ORIENTED_EDGE ( 'NONE', *, *, #14426, .T. ) ;
#10980=PLANE ( 'NONE',  #3897 ) ;
#11009=EDGE_CURVE ( 'NONE', #25398, #9965, #23600, .T. ) ;
#11010=ORIENTED_EDGE ( 'NONE', *, *, #2233, .F. ) ;
#11011=ORIENTED_EDGE ( 'NONE', *, *, #1451, .F. ) ;
#11030=EDGE_CURVE ( 'NONE', #2254, #13002, #11288, .T. ) ;
#11037=CARTESIAN_POINT ( 'NONE',  ( 45.81606138205700063, 34.87886987267150118, 80.75501292736991843 ) ) ;
#11044=ORIENTED_EDGE ( 'NONE', *, *, #23565, .F. ) ;
#11067=EDGE_LOOP ( 'NONE', ( #13119, #5974, #15699, #7040 ) ) ;
#11073=EDGE_CURVE ( 'NONE', #8863, #7140, #11737, .T. ) ;
#11076=DIRECTION ( 'NONE',  ( -6.071532165918830747E-16, 1.000000000000000000, -3.491481338843135327E-15 ) ) ;
#11086=CARTESIAN_POINT ( 'NONE',  ( 44.06606138205700063, 42.11769259596595560, 81.89079936499673806 ) ) ;
#11088=LINE ( 'NONE', #18810, #23613 ) ;
#11092=VECTOR ( 'NONE', #19674, 1000.000000000000000 ) ;
#11098=AXIS2_PLACEMENT_3D ( 'NONE', #19261, #17337, #1721 ) ;
#11112=DIRECTION ( 'NONE',  ( 0.000000000000000000, -1.000000000000000000, 0.000000000000000000 ) ) ;
#11113=CARTESIAN_POINT ( 'NONE',  ( 44.06606138205700063, 40.92314894770294842, 83.08534301325974525 ) ) ;
#11123=ORIENTED_EDGE ( 'NONE', *, *, #11073, .F. ) ;
#11125=LINE ( 'NONE', #6862, #15528 ) ;
#11128=FACE_OUTER_BOUND ( 'NONE', #1924, .T. ) ;
#11140=DIRECTION ( 'NONE',  ( -1.000000000000000000, -1.734723475976814737E-16, 0.000000000000000000 ) ) ;
#11147=EDGE_LOOP ( 'NONE', ( #1463, #20570, #19421, #3007 ) ) ;
#11151=ORIENTED_EDGE ( 'NONE', *, *, #11326, .F. ) ;
#11152=EDGE_CURVE ( 'NONE', #131, #3634, #16327, .T. ) ;
#11162=ADVANCED_FACE ( 'NONE', ( #24304 ), #19957, .F. ) ;
#11166=CYLINDRICAL_SURFACE ( 'NONE', #14170, 10.00000000000000178 ) ;
#11172=CARTESIAN_POINT ( 'NONE',  ( 38.31606138205700063, 0.6124887759231013584, 82.37823623207334833 ) ) ;
#11173=ORIENTED_EDGE ( 'NONE', *, *, #4516, .F. ) ;
#11175=EDGE_CURVE ( 'NONE', #17340, #17183, #19025, .T. ) ;
#11176=CARTESIAN_POINT ( 'NONE',  ( 30.81606138205700418, 0.3928188618129990761, 80.05501292737000085 ) ) ;
#11179=EDGE_LOOP ( 'NONE', ( #18701, #1083, #20957, #17066 ) ) ;
#11181=LINE ( 'NONE', #12988, #3810 ) ;
#11201=AXIS2_PLACEMENT_3D ( 'NONE', #20829, #17222, #14641 ) ;
#11229=LINE ( 'NONE', #4573, #4132 ) ;
#11237=ORIENTED_EDGE ( 'NONE', *, *, #8668, .T. ) ;
#11261=PRODUCT_CONTEXT ( 'NONE', #15387, 'mechanical' ) ;
#11274=VERTEX_POINT ( 'NONE', #18528 ) ;
#11288=CIRCLE ( 'NONE', #12520, 1.500000000000001332 ) ;
#11291=VERTEX_POINT ( 'NONE', #20588 ) ;
#11292=DIRECTION ( 'NONE',  ( 0.000000000000000000, 1.000000000000000000, 0.000000000000000000 ) ) ;
#11301=DIRECTION ( 'NONE',  ( -1.734723475976804876E-16, -3.491481338843135327E-15, -1.000000000000000000 ) ) ;
#11309=LINE ( 'NONE', #24536, #7826 ) ;
#11319=ADVANCED_FACE ( 'NONE', ( #7195 ), #9139, .F. ) ;
#11321=DIRECTION ( 'NONE',  ( 0.000000000000000000, 0.000000000000000000, 1.000000000000000000 ) ) ;
#11322=VERTEX_POINT ( 'NONE', #16985 ) ;
#11326=EDGE_CURVE ( 'NONE', #7039, #3863, #12865, .T. ) ;
#11327=CARTESIAN_POINT ( 'NONE',  ( 35.52536905565747105, -37.40916500673439771, 83.30501292737011454 ) ) ;
#11328=CARTESIAN_POINT ( 'NONE',  ( 35.64099152588522657, 1.142818861812999742, 83.30501292736997243 ) ) ;
#11338=CARTESIAN_POINT ( 'NONE',  ( 44.81606138205700063, 40.39281886181299797, 82.55501292736983032 ) ) ;
#11340=( NAMED_UNIT ( * ) SI_UNIT ( $, .STERADIAN. ) SOLID_ANGLE_UNIT ( ) );
#11341=ORIENTED_EDGE ( 'NONE', *, *, #284, .F. ) ;
#11342=CARTESIAN_POINT ( 'NONE',  ( 40.64099152588522657, -1.357181138186998925, 78.30501292736998664 ) ) ;
#11346=EDGE_LOOP ( 'NONE', ( #1815, #12358, #9014, #8503 ) ) ;
#11347=LINE ( 'NONE', #19431, #9005 ) ;
#11356=EDGE_CURVE ( 'NONE', #23473, #1205, #12997, .T. ) ;
#11367=LINE ( 'NONE', #7881, #8552 ) ;
#11370=DIRECTION ( 'NONE',  ( 0.000000000000000000, -1.000000000000000000, 3.469446951953617344E-15 ) ) ;
#11378=LINE ( 'NONE', #1560, #22917 ) ;
#11385=CARTESIAN_POINT ( 'NONE',  ( 15.14989484155900001, 36.04731275961434989, 84.30501292736985874 ) ) ;
#11390=EDGE_LOOP ( 'NONE', ( #13236, #13431, #3939, #21592 ) ) ;
#11392=ORIENTED_EDGE ( 'NONE', *, *, #5603, .F. ) ;
#11400=DIRECTION ( 'NONE',  ( -1.734723475976814737E-16, -3.009265538105065873E-32, -1.000000000000000000 ) ) ;
#11401=EDGE_LOOP ( 'NONE', ( #21066, #15563, #7107, #11565, #15552, #8118 ) ) ;
#11411=CARTESIAN_POINT ( 'NONE',  ( 40.64099152588522657, 0.3928188618129990761, 80.05501292737000085 ) ) ;
#11427=AXIS2_PLACEMENT_3D ( 'NONE', #19350, #9451, #19472 ) ;
#11464=SURFACE_SIDE_STYLE ('',( #19424 ) ) ;
#11466=DIRECTION ( 'NONE',  ( -1.734723475976804876E-16, -3.469446951953620105E-15, -1.000000000000000000 ) ) ;
#11470=CARTESIAN_POINT ( 'NONE',  ( 31.81606138205700418, -34.67340937580780036, 71.26505871168839690 ) ) ;
#11487=ORIENTED_EDGE ( 'NONE', *, *, #18094, .T. ) ;
#11508=VERTEX_POINT ( 'NONE', #11327 ) ;
#11512=DIRECTION ( 'NONE',  ( -1.510383499235849534E-16, -0.1218693434051499741, -0.9925461516413217611 ) ) ;
#11523=ORIENTED_EDGE ( 'NONE', *, *, #2777, .T. ) ;
#11524=DIRECTION ( 'NONE',  ( 4.336808689942074435E-17, -1.000000000000000000, 3.491481338843135327E-15 ) ) ;
#11527=AXIS2_PLACEMENT_3D ( 'NONE', #22882, #19151, #1487 ) ;
#11530=DIRECTION ( 'NONE',  ( -1.933202721249430383E-16, 0.9925461516413217611, -0.1218693434051499741 ) ) ;
#11537=LINE ( 'NONE', #5851, #10482 ) ;
#11548=FACE_OUTER_BOUND ( 'NONE', #16402, .T. ) ;
#11551=PLANE ( 'NONE',  #15610 ) ;
#11565=ORIENTED_EDGE ( 'NONE', *, *, #13511, .T. ) ;
#11579=CARTESIAN_POINT ( 'NONE',  ( 31.81606138205700418, 24.50429740018177682, 101.9912164131601457 ) ) ;
#11584=DIRECTION ( 'NONE',  ( 1.734723475976814737E-16, 3.009265538105065873E-32, 1.000000000000000000 ) ) ;
#11608=EDGE_LOOP ( 'NONE', ( #6403, #12878, #13789, #10704 ) ) ;
#11620=EDGE_CURVE ( 'NONE', #5274, #13966, #6524, .T. ) ;
#11622=DIRECTION ( 'NONE',  ( -1.000000000000000000, 0.000000000000000000, 1.734723475976804876E-16 ) ) ;
#11632=CARTESIAN_POINT ( 'NONE',  ( 38.31606138205700063, 29.91058581477919986, 95.51211970855651145 ) ) ;
#11647=CIRCLE ( 'NONE', #12056, 0.7500000000000006661 ) ;
#11652=EDGE_LOOP ( 'NONE', ( #14674, #21255, #1098, #15642 ) ) ;
#11663=CIRCLE ( 'NONE', #4244, 3.999999999999899636 ) ;
#11666=CIRCLE ( 'NONE', #10006, 3.000000000000002665 ) ;
#11668=ORIENTED_EDGE ( 'NONE', *, *, #25139, .F. ) ;
#11675=CARTESIAN_POINT ( 'NONE',  ( 42.06606138205700063, 45.04446929126260102, 82.37823623207320622 ) ) ;
#11687=EDGE_CURVE ( 'NONE', #18550, #3395, #12087, .T. ) ;
#11693=AXIS2_PLACEMENT_3D ( 'NONE', #25482, #24747, #7729 ) ;
#11695=LINE ( 'NONE', #19401, #846 ) ;
#11702=ORIENTED_EDGE ( 'NONE', *, *, #22711, .T. ) ;
#11707=CARTESIAN_POINT ( 'NONE',  ( 31.81606138205700418, -36.30035594811090505, 74.91924054225879104 ) ) ;
#11714=ORIENTED_EDGE ( 'NONE', *, *, #15060, .T. ) ;
#11716=LINE ( 'NONE', #19554, #20583 ) ;
#11725=SURFACE_STYLE_USAGE ( .BOTH. , #11464 ) ;
#11731=EDGE_LOOP ( 'NONE', ( #25197, #15301, #8732, #10766 ) ) ;
#11734=CARTESIAN_POINT ( 'NONE',  ( 30.81606138205700418, -38.55876147765410167, 66.30501292737000085 ) ) ;
#11735=EDGE_LOOP ( 'NONE', ( #12583, #25434, #16864, #1360 ) ) ;
#11737=LINE ( 'NONE', #19569, #19845 ) ;
#11742=ORIENTED_EDGE ( 'NONE', *, *, #6714, .F. ) ;
#11751=CARTESIAN_POINT ( 'NONE',  ( 44.06606138205700063, 29.91058581477919986, 95.51211970855651145 ) ) ;
#11752=VECTOR ( 'NONE', #11622, 1000.000000000000000 ) ;
#11754=DIRECTION ( 'NONE',  ( 1.000000000000000000, 1.734723475976804876E-16, -1.734723475976814737E-16 ) ) ;
#11758=ADVANCED_FACE ( 'NONE', ( #21735 ), #11965, .T. ) ;
#11764=FACE_OUTER_BOUND ( 'NONE', #20740, .T. ) ;
#11765=DIRECTION ( 'NONE',  ( -1.000000000000000000, 3.009265538105049890E-31, 1.734723475976809806E-16 ) ) ;
#11770=EDGE_CURVE ( 'NONE', #14052, #17340, #8976, .T. ) ;
#11781=DIRECTION ( 'NONE',  ( 1.734723475976804876E-16, 3.552713678800500140E-15, 1.000000000000000000 ) ) ;
#11792=LINE ( 'NONE', #9725, #19245 ) ;
#11796=DIRECTION ( 'NONE',  ( -1.734723475976814737E-16, 1.000000000000000000, -3.491481338843135327E-15 ) ) ;
#11801=DIRECTION ( 'NONE',  ( 1.000000000000000000, 1.734723475976804876E-16, -1.734723475976814737E-16 ) ) ;
#11807=ORIENTED_EDGE ( 'NONE', *, *, #1948, .T. ) ;
#11818=ORIENTED_EDGE ( 'NONE', *, *, #7366, .F. ) ;
#11822=VECTOR ( 'NONE', #21315, 1000.000000000000000 ) ;
#11828=ORIENTED_EDGE ( 'NONE', *, *, #4831, .F. ) ;
#11849=CYLINDRICAL_SURFACE ( 'NONE', #21915, 10.00000000000000000 ) ;
#11850=SURFACE_SIDE_STYLE ('',( #19690 ) ) ;
#11853=EDGE_LOOP ( 'NONE', ( #8498, #4393, #21970, #6696 ) ) ;
#11855=DIRECTION ( 'NONE',  ( 1.734723475976814737E-16, -1.000000000000000000, 3.491481338843135327E-15 ) ) ;
#11863=LINE ( 'NONE', #12239, #2617 ) ;
#11868=EDGE_CURVE ( 'NONE', #10765, #24723, #13092, .T. ) ;
#11881=CARTESIAN_POINT ( 'NONE',  ( 59.50607210797845426, 32.97469880962110267, 83.30501292736985874 ) ) ;
#11885=PLANE ( 'NONE',  #2041 ) ;
#11911=DIRECTION ( 'NONE',  ( 4.336808689942074435E-17, -1.000000000000000000, 3.491481338843135327E-15 ) ) ;
#11930=CARTESIAN_POINT ( 'NONE',  ( 31.81606138205700418, -27.70293563151089700, 74.66612024218476051 ) ) ;
#11934=CARTESIAN_POINT ( 'NONE',  ( 44.06606138205700063, 40.39281886181299797, 83.30501292736984453 ) ) ;
#11935=ORIENTED_EDGE ( 'NONE', *, *, #2233, .T. ) ;
#11936=VECTOR ( 'NONE', #20382, 1000.000000000000000 ) ;
#11947=DIRECTION ( 'NONE',  ( -5.047295537021760406E-31, 1.000000000000000000, -3.491481338843135327E-15 ) ) ;
#11948=ORIENTED_EDGE ( 'NONE', *, *, #16022, .T. ) ;
#11950=AXIS2_PLACEMENT_3D ( 'NONE', #23584, #13549, #2066 ) ;
#11952=ADVANCED_FACE ( 'NONE', ( #4727, #20433, #3790 ), #15138, .F. ) ;
#11954=CARTESIAN_POINT ( 'NONE',  ( 43.24475484328152675, -1.357181138186998925, 80.05501292736997243 ) ) ;
#11955=CYLINDRICAL_SURFACE ( 'NONE', #6299, 3.999999999999899636 ) ;
#11965=CYLINDRICAL_SURFACE ( 'NONE', #3406, 2.000000000000001776 ) ;
#11969=EDGE_CURVE ( 'NONE', #643, #16610, #24365, .T. ) ;
#11981=DIRECTION ( 'NONE',  ( 1.734723475976814737E-16, -1.000000000000000000, 3.491481338843135327E-15 ) ) ;
#11984=ORIENTED_EDGE ( 'NONE', *, *, #18533, .F. ) ;
#11997=ORIENTED_EDGE ( 'NONE', *, *, #13973, .T. ) ;
#12011=CARTESIAN_POINT ( 'NONE',  ( 40.64099152588523367, -8.607181138186998481, 88.30501292736998664 ) ) ;
#12049=CARTESIAN_POINT ( 'NONE',  ( 35.64099152588522657, -8.167181138186998979, 78.30501292736998664 ) ) ;
#12050=DIRECTION ( 'NONE',  ( -1.000000000000000000, 4.930380657631319405E-32, 1.734723475976804876E-16 ) ) ;
#12056=AXIS2_PLACEMENT_3D ( 'NONE', #3086, #22920, #885 ) ;
#12079=DIRECTION ( 'NONE',  ( 1.000000000000000000, 2.065146995210479765E-16, -1.734723475976814737E-16 ) ) ;
#12085=CARTESIAN_POINT ( 'NONE',  ( 35.64099152588522657, 0.3928188618129990761, 82.55501292736997243 ) ) ;
#12087=LINE ( 'NONE', #2648, #924 ) ;
#12088=DIRECTION ( 'NONE',  ( -1.734723475976804876E-16, -3.491481338843135327E-15, -1.000000000000000000 ) ) ;
#12122=LINE ( 'NONE', #7731, #18280 ) ;
#12127=DIRECTION ( 'NONE',  ( 1.000000000000000000, 1.734723475976804876E-16, -1.734723475976814737E-16 ) ) ;
#12129=ORIENTED_EDGE ( 'NONE', *, *, #13692, .F. ) ;
#12133=EDGE_CURVE ( 'NONE', #7783, #4335, #11663, .T. ) ;
#12136=ORIENTED_EDGE ( 'NONE', *, *, #15538, .F. ) ;
#12145=CARTESIAN_POINT ( 'NONE',  ( 32.56606138205700773, 47.04446929126254417, 81.37823623207319201 ) ) ;
#12157=VECTOR ( 'NONE', #22280, 1000.000000000000000 ) ;
#12174=DIRECTION ( 'NONE',  ( 0.000000000000000000, 0.7071067811865427988, 0.7071067811865521247 ) ) ;
#12197=EDGE_LOOP ( 'NONE', ( #19024, #11173, #23077, #21873 ) ) ;
#12200=DIRECTION ( 'NONE',  ( 1.000000000000000000, 1.734723475976814737E-16, -1.734723475976809806E-16 ) ) ;
#12210=CARTESIAN_POINT ( 'NONE',  ( 40.64099152588523367, 1.392818861812999964, 93.30501292736998664 ) ) ;
#12221=DIRECTION ( 'NONE',  ( 0.000000000000000000, 1.000000000000000000, -3.304235192336775512E-15 ) ) ;
#12231=ADVANCED_FACE ( 'NONE', ( #23751 ), #10235, .F. ) ;
#12234=EDGE_CURVE ( 'NONE', #22820, #3395, #4439, .T. ) ;
#12239=CARTESIAN_POINT ( 'NONE',  ( 44.81606138205700063, -26.74044063519535186, 82.55501292737007191 ) ) ;
#12242=EDGE_LOOP ( 'NONE', ( #5562, #2502, #10521, #19400, #22180, #4185, #7778, #16065 ) ) ;
#12246=ORIENTED_EDGE ( 'NONE', *, *, #994, .T. ) ;
#12251=AXIS2_PLACEMENT_3D ( 'NONE', #14966, #5185, #13039 ) ;
#12252=CIRCLE ( 'NONE', #6891, 1.750000000000001554 ) ;
#12292=CARTESIAN_POINT ( 'NONE',  ( 30.81606138205700418, 0.3928188618129990761, 82.55501292736998664 ) ) ;
#12300=VERTEX_POINT ( 'NONE', #16662 ) ;
#12321=ADVANCED_FACE ( 'NONE', ( #24753 ), #18727, .F. ) ;
#12325=ORIENTED_EDGE ( 'NONE', *, *, #2054, .F. ) ;
#12326=CARTESIAN_POINT ( 'NONE',  ( 45.81606138205700063, -30.95005513552129983, 81.04249030099066431 ) ) ;
#12339=EDGE_CURVE ( 'NONE', #5120, #17340, #805, .T. ) ;
#12347=CARTESIAN_POINT ( 'NONE',  ( 44.06606138205700063, 45.04446929126260102, 82.37823623207320622 ) ) ;
#12355=VECTOR ( 'NONE', #15901, 1000.000000000000000 ) ;
#12356=EDGE_CURVE ( 'NONE', #13535, #9362, #18592, .T. ) ;
#12357=ORIENTED_EDGE ( 'NONE', *, *, #6812, .F. ) ;
#12358=ORIENTED_EDGE ( 'NONE', *, *, #14230, .T. ) ;
#12359=PLANE ( 'NONE',  #2947 ) ;
#12378=ORIENTED_EDGE ( 'NONE', *, *, #23502, .T. ) ;
#12384=FACE_OUTER_BOUND ( 'NONE', #11853, .T. ) ;
#12398=LINE ( 'NONE', #22291, #7725 ) ;
#12406=DIRECTION ( 'NONE',  ( 1.000000000000000000, 1.734723475976804876E-16, -1.734723475976814737E-16 ) ) ;
#12411=EDGE_LOOP ( 'NONE', ( #8282, #13107, #18721, #22929 ) ) ;
#12415=AXIS2_PLACEMENT_3D ( 'NONE', #16806, #8961, #14370 ) ;
#12419=ORIENTED_EDGE ( 'NONE', *, *, #9650, .F. ) ;
#12427=EDGE_CURVE ( 'NONE', #24509, #23758, #20791, .T. ) ;
#12429=EDGE_CURVE ( 'NONE', #9362, #2551, #3383, .T. ) ;
#12433=DIRECTION ( 'NONE',  ( -1.000000000000000000, -1.734723475976804876E-16, 1.734723475976814737E-16 ) ) ;
#12458=VECTOR ( 'NONE', #7439, 1000.000000000000000 ) ;
#12467=DIRECTION ( 'NONE',  ( 1.734723475976805122E-16, -1.000000000000000000, 0.000000000000000000 ) ) ;
#12477=DIRECTION ( 'NONE',  ( -1.734723475976804876E-16, -3.491481338843135327E-15, -1.000000000000000000 ) ) ;
#12492=VECTOR ( 'NONE', #11781, 1000.000000000000000 ) ;
#12496=CARTESIAN_POINT ( 'NONE',  ( 31.81606138205700418, -36.30035594811090505, 74.91924054225879104 ) ) ;
#12497=VECTOR ( 'NONE', #661, 1000.000000000000000 ) ;
#12504=ADVANCED_FACE ( 'NONE', ( #11128 ), #1563, .T. ) ;
#12510=ORIENTED_EDGE ( 'NONE', *, *, #15871, .T. ) ;
#12511=ORIENTED_EDGE ( 'NONE', *, *, #4827, .T. ) ;
#12520=AXIS2_PLACEMENT_3D ( 'NONE', #23685, #5322, #13904 ) ;
#12522=FACE_OUTER_BOUND ( 'NONE', #1862, .T. ) ;
#12533=DIRECTION ( 'NONE',  ( 0.000000000000000000, -1.000000000000000000, 0.000000000000000000 ) ) ;
#12539=DIRECTION ( 'NONE',  ( -1.734723475976804876E-16, -3.491481338843135327E-15, -1.000000000000000000 ) ) ;
#12550=EDGE_LOOP ( 'NONE', ( #24145, #10406, #5747, #7922 ) ) ;
#12557=DIRECTION ( 'NONE',  ( 1.734723475976804876E-16, 3.496552006265755350E-15, 1.000000000000000000 ) ) ;
#12560=VERTEX_POINT ( 'NONE', #21415 ) ;
#12564=PLANE ( 'NONE',  #1102 ) ;
#12583=ORIENTED_EDGE ( 'NONE', *, *, #12356, .F. ) ;
#12591=VERTEX_POINT ( 'NONE', #8140 ) ;
#12596=LINE ( 'NONE', #4971, #3201 ) ;
#12601=CARTESIAN_POINT ( 'NONE',  ( 34.56606138205700773, 47.04446929126260102, 82.37823623207320622 ) ) ;
#12606=EDGE_LOOP ( 'NONE', ( #724, #20535, #19282, #16425 ) ) ;
#12620=DIRECTION ( 'NONE',  ( 0.000000000000000000, 1.000000000000000000, -3.469446951953614189E-15 ) ) ;
#12656=EDGE_LOOP ( 'NONE', ( #12378, #9469, #15312, #25448 ) ) ;
#12660=AXIS2_PLACEMENT_3D ( 'NONE', #13382, #21226, #19285 ) ;
#12662=ORIENTED_EDGE ( 'NONE', *, *, #9650, .T. ) ;
#12680=AXIS2_PLACEMENT_3D ( 'NONE', #16111, #8883, #14791 ) ;
#12688=CARTESIAN_POINT ( 'NONE',  ( 35.64099152588522657, 1.142818861812999742, 82.55501292736997243 ) ) ;
#12715=ORIENTED_EDGE ( 'NONE', *, *, #7939, .T. ) ;
#12725=ORIENTED_EDGE ( 'NONE', *, *, #584, .F. ) ;
#12729=EDGE_CURVE ( 'NONE', #14052, #24921, #21543, .T. ) ;
#12734=FACE_OUTER_BOUND ( 'NONE', #12656, .T. ) ;
#12738=EDGE_CURVE ( 'NONE', #20175, #2245, #4678, .T. ) ;
#12747=DIRECTION ( 'NONE',  ( 1.000000000000000000, 1.734723475976804876E-16, -1.734723475976814737E-16 ) ) ;
#12748=ADVANCED_FACE ( 'NONE', ( #6834 ), #20757, .F. ) ;
#12755=ORIENTED_EDGE ( 'NONE', *, *, #13102, .F. ) ;
#12766=DIRECTION ( 'NONE',  ( 0.000000000000000000, 0.000000000000000000, 1.000000000000000000 ) ) ;
#12769=DIRECTION ( 'NONE',  ( 1.734723475976814737E-16, 0.000000000000000000, 1.000000000000000000 ) ) ;
#12779=DIRECTION ( 'NONE',  ( 0.000000000000000000, 1.000000000000000000, -4.625929269271481378E-15 ) ) ;
#12783=LINE ( 'NONE', #10843, #2028 ) ;
#12794=AXIS2_PLACEMENT_3D ( 'NONE', #12326, #10255, #21972 ) ;
#12797=FACE_OUTER_BOUND ( 'NONE', #218, .T. ) ;
#12801=DIRECTION ( 'NONE',  ( 1.000000000000000000, -3.009265538105074850E-31, -1.734723475976809806E-16 ) ) ;
#12809=DIRECTION ( 'NONE',  ( -1.000000000000000000, -1.734723475976814737E-16, 8.024708101613549867E-31 ) ) ;
#12819=ORIENTED_EDGE ( 'NONE', *, *, #21686, .F. ) ;
#12820=DIRECTION ( 'NONE',  ( -1.734723475976804876E-16, 1.000000000000000000, 0.000000000000000000 ) ) ;
#12841=DIRECTION ( 'NONE',  ( -1.000000000000000000, -1.734723475976804876E-16, 1.734723475976814737E-16 ) ) ;
#12842=DIRECTION ( 'NONE',  ( 1.734723475976804876E-16, -1.000000000000000000, -3.009265538105065326E-32 ) ) ;
#12845=FACE_OUTER_BOUND ( 'NONE', #11401, .T. ) ;
#12856=DIRECTION ( 'NONE',  ( -8.791731484610113542E-17, 0.9135454576426023099, 0.4067366430757970996 ) ) ;
#12859=DIRECTION ( 'NONE',  ( 0.000000000000000000, 0.000000000000000000, 1.000000000000000000 ) ) ;
#12865=LINE ( 'NONE', #3184, #9161 ) ;
#12870=AXIS2_PLACEMENT_3D ( 'NONE', #16165, #12200, #21973 ) ;
#12871=EDGE_CURVE ( 'NONE', #25303, #10220, #6734, .T. ) ;
#12878=ORIENTED_EDGE ( 'NONE', *, *, #22491, .T. ) ;
#12881=UNCERTAINTY_MEASURE_WITH_UNIT (LENGTH_MEASURE( 1.000000000000000082E-05 ), #19182, 'distance_accuracy_value', 'NONE');
#12903=EDGE_CURVE ( 'NONE', #17183, #18894, #17264, .T. ) ;
#12912=DIRECTION ( 'NONE',  ( 0.000000000000000000, -3.491481338843135327E-15, -1.000000000000000000 ) ) ;
#12922=CARTESIAN_POINT ( 'NONE',  ( 44.06606138205700063, 40.39281886181299797, 82.55501292736983032 ) ) ;
#12946=ORIENTED_EDGE ( 'NONE', *, *, #9081, .T. ) ;
#12949=CARTESIAN_POINT ( 'NONE',  ( 44.81606138205700063, -26.97987052895604876, 80.55501292737007191 ) ) ;
#12987=ORIENTED_EDGE ( 'NONE', *, *, #14602, .T. ) ;
#12988=CARTESIAN_POINT ( 'NONE',  ( 35.64099152588523367, -8.607181138186998481, 88.30501292736998664 ) ) ;
#12997=LINE ( 'NONE', #22894, #7100 ) ;
#12999=FACE_OUTER_BOUND ( 'NONE', #11652, .T. ) ;
#13000=EDGE_CURVE ( 'NONE', #10641, #12591, #15325, .T. ) ;
#13002=VERTEX_POINT ( 'NONE', #3596 ) ;
#13006=ORIENTED_EDGE ( 'NONE', *, *, #12429, .T. ) ;
#13016=EDGE_CURVE ( 'NONE', #4112, #14925, #16200, .T. ) ;
#13039=DIRECTION ( 'NONE',  ( 0.000000000000000000, 1.000000000000000000, 0.000000000000000000 ) ) ;
#13043=LINE ( 'NONE', #24356, #16187 ) ;
#13073=PLANE ( 'NONE',  #516 ) ;
#13088=CARTESIAN_POINT ( 'NONE',  ( 32.56606138205700773, 41.63025572888945192, 83.79244979444629848 ) ) ;
#13092=LINE ( 'NONE', #20944, #21519 ) ;
#13097=EDGE_CURVE ( 'NONE', #10140, #4783, #17852, .T. ) ;
#13102=EDGE_CURVE ( 'NONE', #8461, #4335, #12122, .T. ) ;
#13106=LINE ( 'NONE', #972, #8695 ) ;
#13107=ORIENTED_EDGE ( 'NONE', *, *, #261, .T. ) ;
#13119=ORIENTED_EDGE ( 'NONE', *, *, #3014, .F. ) ;
#13120=AXIS2_PLACEMENT_3D ( 'NONE', #6649, #2896, #4843 ) ;
#13160=EDGE_LOOP ( 'NONE', ( #2481, #19378, #20799, #15023 ) ) ;
#13173=DIRECTION ( 'NONE',  ( 1.000000000000000000, 1.734723475976804876E-16, -1.734723475976814737E-16 ) ) ;
#13175=EDGE_CURVE ( 'NONE', #2290, #6422, #110, .T. ) ;
#13189=EDGE_CURVE ( 'NONE', #17064, #17020, #11863, .T. ) ;
#13203=CYLINDRICAL_SURFACE ( 'NONE', #938, 1.750000000000001554 ) ;
#13207=VERTEX_POINT ( 'NONE', #9116 ) ;
#13211=EDGE_CURVE ( 'NONE', #8863, #2531, #22745, .T. ) ;
#13218=ORIENTED_EDGE ( 'NONE', *, *, #574, .F. ) ;
#13220=CARTESIAN_POINT ( 'NONE',  ( 40.64099152588522657, 1.392818861812999964, 83.30501292736997243 ) ) ;
#13223=ADVANCED_FACE ( 'NONE', ( #2548 ), #11166, .T. ) ;
#13229=CYLINDRICAL_SURFACE ( 'NONE', #14737, 0.7500000000000006661 ) ;
#13234=DIRECTION ( 'NONE',  ( 1.734723475976804876E-16, 3.469446951953610245E-15, 1.000000000000000000 ) ) ;
#13236=ORIENTED_EDGE ( 'NONE', *, *, #25171, .T. ) ;
#13247=CARTESIAN_POINT ( 'NONE',  ( 32.56606138205700773, -26.74044063519535186, 83.30501292737007191 ) ) ;
#13251=FACE_OUTER_BOUND ( 'NONE', #10262, .T. ) ;
#13261=ORIENTED_EDGE ( 'NONE', *, *, #15385, .T. ) ;
#13270=ORIENTED_EDGE ( 'NONE', *, *, #21999, .F. ) ;
#13285=ORIENTED_EDGE ( 'NONE', *, *, #16, .T. ) ;
#13296=VERTEX_POINT ( 'NONE', #2422 ) ;
#13299=CARTESIAN_POINT ( 'NONE',  ( 32.56606138205700773, 0.6124887759231013584, 82.37823623207334833 ) ) ;
#13308=CARTESIAN_POINT ( 'NONE',  ( 32.56606138205700773, 42.11769259596595560, 81.89079936499675227 ) ) ;
#13341=EDGE_CURVE ( 'NONE', #2117, #21490, #18292, .T. ) ;
#13344=EDGE_CURVE ( 'NONE', #17183, #24921, #3032, .T. ) ;
#13354=FACE_OUTER_BOUND ( 'NONE', #7426, .T. ) ;
#13382=CARTESIAN_POINT ( 'NONE',  ( 32.56606138205700773, 43.35512946304240245, 83.12823623207320622 ) ) ;
#13386=CARTESIAN_POINT ( 'NONE',  ( 31.81606138205700418, 34.87886987267149408, 80.75501292736991843 ) ) ;
#13397=CARTESIAN_POINT ( 'NONE',  ( 31.81606138205700418, 40.39281886181299797, 80.75501292736983316 ) ) ;
#13417=EDGE_LOOP ( 'NONE', ( #14250, #19788, #22232, #11818 ) ) ;
#13429=EDGE_CURVE ( 'NONE', #18894, #11508, #19664, .T. ) ;
#13431=ORIENTED_EDGE ( 'NONE', *, *, #15725, .T. ) ;
#13442=ORIENTED_EDGE ( 'NONE', *, *, #2654, .T. ) ;
#13450=DIRECTION ( 'NONE',  ( 1.000000000000000000, 6.071532165918830747E-16, -1.734723475976829774E-16 ) ) ;
#13457=VECTOR ( 'NONE', #9490, 1000.000000000000000 ) ;
#13460=AXIS2_PLACEMENT_3D ( 'NONE', #11632, #9823, #17678 ) ;
#13462=DIRECTION ( 'NONE',  ( -1.000000000000000000, -2.168404344971055214E-16, 1.734723475976814737E-16 ) ) ;
#13473=CARTESIAN_POINT ( 'NONE',  ( 38.41621794735363693, -36.60729675983900222, 83.30501292737011454 ) ) ;
#13492=VERTEX_POINT ( 'NONE', #17875 ) ;
#13510=ADVANCED_FACE ( 'NONE', ( #15802 ), #11955, .T. ) ;
#13511=EDGE_CURVE ( 'NONE', #22911, #21429, #7994, .T. ) ;
#13515=( NAMED_UNIT ( * ) SI_UNIT ( $, .STERADIAN. ) SOLID_ANGLE_UNIT ( ) );
#13535=VERTEX_POINT ( 'NONE', #19913 ) ;
#13543=CIRCLE ( 'NONE', #18897, 1.750000000000001554 ) ;
#13545=ORIENTED_EDGE ( 'NONE', *, *, #10524, .T. ) ;
#13546=CARTESIAN_POINT ( 'NONE',  ( 30.81606138205700418, -0.6071811381869983704, 80.05501292737000085 ) ) ;
#13547=DIRECTION ( 'NONE',  ( 1.734723475976814737E-16, -1.000000000000000000, 3.491481338843135327E-15 ) ) ;
#13549=DIRECTION ( 'NONE',  ( 2.595751990468335074E-30, 1.000000000000000000, -3.491481338843135327E-15 ) ) ;
#13588=ORIENTED_EDGE ( 'NONE', *, *, #11356, .T. ) ;
#13609=ORIENTED_EDGE ( 'NONE', *, *, #21858, .T. ) ;
#13637=VECTOR ( 'NONE', #8198, 1000.000000000000000 ) ;
#13644=CARTESIAN_POINT ( 'NONE',  ( 42.06606138205700063, 47.04446929126260102, 82.37823623207320622 ) ) ;
#13648=CARTESIAN_POINT ( 'NONE',  ( 35.64099152588522657, 1.392818861812999964, 84.30501292737000085 ) ) ;
#13649=LINE ( 'NONE', #101, #1743 ) ;
#13668=EDGE_LOOP ( 'NONE', ( #6878, #18709, #5913, #16967 ) ) ;
#13676=CIRCLE ( 'NONE', #24331, 12.59999999999999964 ) ;
#13678=DIRECTION ( 'NONE',  ( -1.809068767804384992E-15, -1.000000000000000000, 3.491481338843135327E-15 ) ) ;
#13692=EDGE_CURVE ( 'NONE', #7151, #16594, #2219, .T. ) ;
#13706=DIRECTION ( 'NONE',  ( 0.000000000000000000, -1.000000000000000000, 6.123233995736769734E-17 ) ) ;
#13716=ORIENTED_EDGE ( 'NONE', *, *, #17120, .F. ) ;
#13731=LINE ( 'NONE', #5611, #7866 ) ;
#13761=LINE ( 'NONE', #17751, #24190 ) ;
#13767=ORIENTED_EDGE ( 'NONE', *, *, #17059, .F. ) ;
#13777=ORIENTED_EDGE ( 'NONE', *, *, #24087, .T. ) ;
#13778=CARTESIAN_POINT ( 'NONE',  ( 44.81606138205700063, -38.55876147765410167, 72.21586839016146087 ) ) ;
#13789=ORIENTED_EDGE ( 'NONE', *, *, #11073, .T. ) ;
#13806=EDGE_CURVE ( 'NONE', #19200, #2551, #5085, .T. ) ;
#13814=ADVANCED_FACE ( 'NONE', ( #10762 ), #13073, .F. ) ;
#13818=ORIENTED_EDGE ( 'NONE', *, *, #13000, .T. ) ;
#13821=LINE ( 'NONE', #25136, #1228 ) ;
#13825=ADVANCED_FACE ( 'NONE', ( #4951 ), #13203, .T. ) ;
#13826=EDGE_CURVE ( 'NONE', #6661, #21036, #18233, .T. ) ;
#13841=DIRECTION ( 'NONE',  ( 0.000000000000000000, -1.000000000000000000, 0.000000000000000000 ) ) ;
#13849=CARTESIAN_POINT ( 'NONE',  ( 35.64099152588522657, -9.607181138187000258, 73.02501292736999972 ) ) ;
#13852=DIRECTION ( 'NONE',  ( 0.000000000000000000, -1.000000000000000000, 3.491481338843135327E-15 ) ) ;
#13856=EDGE_LOOP ( 'NONE', ( #7810, #12510, #585, #11487 ) ) ;
#13863=CARTESIAN_POINT ( 'NONE',  ( 44.06606138205700063, 40.39281886181299797, 82.55501292736983032 ) ) ;
#13870=CARTESIAN_POINT ( 'NONE',  ( 45.81606138205700063, -36.30035594811079847, 74.91924054225879104 ) ) ;
#13886=AXIS2_PLACEMENT_3D ( 'NONE', #8747, #6549, #12620 ) ;
#13888=FACE_OUTER_BOUND ( 'NONE', #16221, .T. ) ;
#13890=ORIENTED_EDGE ( 'NONE', *, *, #19571, .F. ) ;
#13898=VECTOR ( 'NONE', #21740, 1000.000000000000000 ) ;
#13904=DIRECTION ( 'NONE',  ( 0.000000000000000000, 1.000000000000000000, 0.000000000000000000 ) ) ;
#13913=DIRECTION ( 'NONE',  ( -5.047295537021760406E-31, 1.000000000000000000, -3.491481338843135327E-15 ) ) ;
#13915=CIRCLE ( 'NONE', #6503, 1.000000000000000888 ) ;
#13927=ORIENTED_EDGE ( 'NONE', *, *, #8829, .T. ) ;
#13928=PLANE ( 'NONE',  #6806 ) ;
#13947=VERTEX_POINT ( 'NONE', #17567 ) ;
#13956=CARTESIAN_POINT ( 'NONE',  ( 40.64099152588522657, -9.607181138187000258, 82.55501292736997243 ) ) ;
#13966=VERTEX_POINT ( 'NONE', #9595 ) ;
#13973=EDGE_CURVE ( 'NONE', #13207, #18741, #7652, .T. ) ;
#13982=CARTESIAN_POINT ( 'NONE',  ( 30.81606138205700418, 40.39281886181299797, 66.30501292737000085 ) ) ;
#13997=LINE ( 'NONE', #21846, #18162 ) ;
#13998=VECTOR ( 'NONE', #15974, 1000.000000000000000 ) ;
#14003=CARTESIAN_POINT ( 'NONE',  ( 30.81606138205700418, -3.831401139557048197, 80.75501292737000369 ) ) ;
#14012=PLANE ( 'NONE',  #3668 ) ;
#14013=CARTESIAN_POINT ( 'NONE',  ( 45.81606138205700063, -36.05876147765410877, 70.30501292737000085 ) ) ;
#14027=VERTEX_POINT ( 'NONE', #17696 ) ;
#14029=EDGE_CURVE ( 'NONE', #24723, #22752, #7121, .T. ) ;
#14049=ADVANCED_FACE ( 'NONE', ( #7524 ), #15372, .T. ) ;
#14052=VERTEX_POINT ( 'NONE', #21935 ) ;
#14071=VECTOR ( 'NONE', #18522, 1000.000000000000000 ) ;
#14072=VECTOR ( 'NONE', #18024, 1000.000000000000000 ) ;
#14074=DIRECTION ( 'NONE',  ( 1.000000000000000000, 1.734723475976804876E-16, -1.734723475976814737E-16 ) ) ;
#14090=DIRECTION ( 'NONE',  ( 1.734723475976739795E-16, 4.343580702399009298E-14, 1.000000000000000000 ) ) ;
#14095=EDGE_CURVE ( 'NONE', #10641, #3863, #19058, .T. ) ;
#14096=AXIS2_PLACEMENT_3D ( 'NONE', #983, #19155, #8871 ) ;
#14099=DIRECTION ( 'NONE',  ( 1.000000000000000000, 2.168404344971050037E-16, -1.734723475976814737E-16 ) ) ;
#14104=FACE_OUTER_BOUND ( 'NONE', #13160, .T. ) ;
#14121=CIRCLE ( 'NONE', #2581, 3.999999999999899636 ) ;
#14136=DIRECTION ( 'NONE',  ( -1.000000000000000000, -2.168404344971010101E-16, 1.734723475976814737E-16 ) ) ;
#14143=DIRECTION ( 'NONE',  ( -1.000000000000000000, 6.018531076210130433E-31, 1.734723475976804876E-16 ) ) ;
#14147=ORIENTED_EDGE ( 'NONE', *, *, #11030, .F. ) ;
#14148=CARTESIAN_POINT ( 'NONE',  ( 45.81606138205700063, -34.55876147765410167, 70.30501292737000085 ) ) ;
#14157=AXIS2_PLACEMENT_3D ( 'NONE', #22676, #24207, #10840 ) ;
#14166=DIRECTION ( 'NONE',  ( -1.734723475976804876E-16, -3.469446951953610245E-15, -1.000000000000000000 ) ) ;
#14170=AXIS2_PLACEMENT_3D ( 'NONE', #22874, #16827, #18889 ) ;
#14204=ADVANCED_FACE ( 'NONE', ( #24946 ), #15179, .F. ) ;
#14211=VERTEX_POINT ( 'NONE', #22908 ) ;
#14213=VERTEX_POINT ( 'NONE', #11338 ) ;
#14225=LINE ( 'NONE', #2479, #21715 ) ;
#14230=EDGE_CURVE ( 'NONE', #6270, #7648, #1402, .T. ) ;
#14245=EDGE_LOOP ( 'NONE', ( #4179, #20414, #12136, #5591, #18676, #493, #11668, #20290 ) ) ;
#14250=ORIENTED_EDGE ( 'NONE', *, *, #11620, .F. ) ;
#14262=FACE_OUTER_BOUND ( 'NONE', #11608, .T. ) ;
#14268=ORIENTED_EDGE ( 'NONE', *, *, #15712, .F. ) ;
#14283=VECTOR ( 'NONE', #21419, 1000.000000000000000 ) ;
#14322=ORIENTED_EDGE ( 'NONE', *, *, #12356, .T. ) ;
#14325=PLANE ( 'NONE',  #6050 ) ;
#14344=VECTOR ( 'NONE', #15322, 1000.000000000000000 ) ;
#14360=ORIENTED_EDGE ( 'NONE', *, *, #8885, .T. ) ;
#14367=ORIENTED_EDGE ( 'NONE', *, *, #6273, .F. ) ;
#14370=DIRECTION ( 'NONE',  ( -1.734723475976814737E-16, 0.000000000000000000, -1.000000000000000000 ) ) ;
#14378=ORIENTED_EDGE ( 'NONE', *, *, #6714, .T. ) ;
#14387=AXIS2_PLACEMENT_3D ( 'NONE', #5391, #19168, #7836 ) ;
#14426=EDGE_CURVE ( 'NONE', #18741, #6360, #5780, .T. ) ;
#14430=CARTESIAN_POINT ( 'NONE',  ( 31.81606138205700418, 40.39281886181299797, 66.30501292737000085 ) ) ;
#14439=AXIS2_PLACEMENT_3D ( 'NONE', #10567, #752, #8638 ) ;
#14443=EDGE_CURVE ( 'NONE', #4268, #9258, #4235, .T. ) ;
#14471=CARTESIAN_POINT ( 'NONE',  ( 30.81606138205700418, -11.72563467517899838, 72.98595903681224684 ) ) ;
#14481=LINE ( 'NONE', #18353, #17998 ) ;
#14511=VECTOR ( 'NONE', #22870, 1000.000000000000000 ) ;
#14513=LINE ( 'NONE', #7172, #21369 ) ;
#14515=ADVANCED_FACE ( 'NONE', ( #8099 ), #15942, .F. ) ;
#14519=ORIENTED_EDGE ( 'NONE', *, *, #22711, .F. ) ;
#14581=CARTESIAN_POINT ( 'NONE',  ( 35.64099152588522657, 1.142818861812999742, 84.30501292737000085 ) ) ;
#14583=CARTESIAN_POINT ( 'NONE',  ( 38.41621794735363693, -38.10729675983899511, 83.30501292737011454 ) ) ;
#14585=ADVANCED_FACE ( 'NONE', ( #16071 ), #725, .F. ) ;
#14589=CARTESIAN_POINT ( 'NONE',  ( 32.56606138205700773, 40.39281886181299797, 83.30501292736984453 ) ) ;
#14602=EDGE_CURVE ( 'NONE', #13002, #2254, #23108, .T. ) ;
#14603=CARTESIAN_POINT ( 'NONE',  ( 44.06606138205700063, 0.6124887759231013584, 82.37823623207334833 ) ) ;
#14613=DIRECTION ( 'NONE',  ( 0.000000000000000000, 1.000000000000000000, 0.000000000000000000 ) ) ;
#14633=CARTESIAN_POINT ( 'NONE',  ( 31.81606138205700418, -34.55876147765410167, 70.30501292737000085 ) ) ;
#14636=CARTESIAN_POINT ( 'NONE',  ( 35.64099152588522657, -0.6071811381869983704, 80.05501292737000085 ) ) ;
#14641=DIRECTION ( 'NONE',  ( 0.000000000000000000, 1.000000000000000000, 0.000000000000000000 ) ) ;
#14643=LINE ( 'NONE', #18768, #9066 ) ;
#14650=CARTESIAN_POINT ( 'NONE',  ( 17.31606138205699708, 34.87886987267149408, 81.44836866983821722 ) ) ;
#14654=DIRECTION ( 'NONE',  ( -1.734723475976804876E-16, -3.430248998885765387E-15, -1.000000000000000000 ) ) ;
#14658=FACE_OUTER_BOUND ( 'NONE', #5102, .T. ) ;
#14667=FACE_OUTER_BOUND ( 'NONE', #16778, .T. ) ;
#14669=ORIENTED_EDGE ( 'NONE', *, *, #17940, .T. ) ;
#14673=VECTOR ( 'NONE', #24398, 1000.000000000000000 ) ;
#14674=ORIENTED_EDGE ( 'NONE', *, *, #13973, .F. ) ;
#14675=ADVANCED_FACE ( 'NONE', ( #12734 ), #12359, .F. ) ;
#14677=FACE_OUTER_BOUND ( 'NONE', #20553, .T. ) ;
#14682=DIRECTION ( 'NONE',  ( 0.000000000000000000, -3.491481338843135327E-15, -1.000000000000000000 ) ) ;
#14684=SHAPE_REPRESENTATION ( 'Metal Base Plate', ( #2000 ), #15777 ) ;
#14692=EDGE_LOOP ( 'NONE', ( #1045, #654, #6406, #15415, #20632, #11392, #24441, #19030, #16295, #9505, #8389, #9549, #10002, #6271, #6827, #6843 ) ) ;
#14693=CLOSED_SHELL ( 'NONE', ( #24691, #24352, #20613, #3802, #16174, #7697, #13825, #4618, #6659, #24047, #19715, #4025, #7532, #23233, #8238, #22772, #23024, #13814, #16463, #10835, #5477, #394, #2019, #17660, #14049, #13223, #4689, #16189, #3720, #14515, #3761, #7132, #6120, #10931, #19175, #13510, #12231, #18882, #18585, #18232, #10466, #15527, #11319, #12748, #11162, #2292, #7987, #22247, #6579, #4428, #10518, #9913, #10677, #11758, #10291, #17475, #24493, #19663, #25205, #2330, #12321, #4979, #6458, #10917, #5558, #2020, #14585, #6485, #1675, #15068, #10836, #19869, #8783, #18490, #24268, #9276, #14785, #2605, #19293, #16390, #21848, #12504, #21374, #21866, #6809, #8803, #4463, #10331, #19008, #11952, #22961, #15847, #10453, #7923, #14675, #10366, #14204, #16358 ) ) ;
#14697=AXIS2_PLACEMENT_3D ( 'NONE', #3693, #1622, #19410 ) ;
#14715=EDGE_LOOP ( 'NONE', ( #14873, #15316, #24345, #12725 ) ) ;
#14734=CARTESIAN_POINT ( 'NONE',  ( 38.41621794735363693, -36.60729675983900222, 84.30501292737011454 ) ) ;
#14737=AXIS2_PLACEMENT_3D ( 'NONE', #23117, #22995, #19518 ) ;
#14750=ORIENTED_EDGE ( 'NONE', *, *, #10524, .F. ) ;
#14756=CYLINDRICAL_SURFACE ( 'NONE', #21929, 2.000000000000001776 ) ;
#14760=AXIS2_PLACEMENT_3D ( 'NONE', #8179, #17719, #4320 ) ;
#14785=ADVANCED_FACE ( 'NONE', ( #5248 ), #17227, .T. ) ;
#14789=VECTOR ( 'NONE', #4353, 1000.000000000000000 ) ;
#14791=DIRECTION ( 'NONE',  ( -1.734723475976804876E-16, 1.000000000000000000, 0.000000000000000000 ) ) ;
#14792=DIRECTION ( 'NONE',  ( -1.734723475976804876E-16, -3.469446951953610245E-15, -1.000000000000000000 ) ) ;
#14794=ORIENTED_EDGE ( 'NONE', *, *, #23908, .T. ) ;
#14804=DIRECTION ( 'NONE',  ( -8.791731484610113542E-17, 0.9135454576426023099, 0.4067366430757970996 ) ) ;
#14823=EDGE_CURVE ( 'NONE', #18487, #2496, #14900, .T. ) ;
#14837=DIRECTION ( 'NONE',  ( -1.734723475976804876E-16, -3.269436733918100469E-15, -1.000000000000000000 ) ) ;
#14864=LINE ( 'NONE', #22726, #21982 ) ;
#14866=ORIENTED_EDGE ( 'NONE', *, *, #9499, .F. ) ;
#14872=ORIENTED_EDGE ( 'NONE', *, *, #22638, .F. ) ;
#14873=ORIENTED_EDGE ( 'NONE', *, *, #22810, .F. ) ;
#14881=DIRECTION ( 'NONE',  ( -1.000000000000000000, -1.734723475976804876E-16, 1.734723475976814737E-16 ) ) ;
#14889=CARTESIAN_POINT ( 'NONE',  ( 35.64099152588522657, -8.607181138186998481, 79.30501292737000085 ) ) ;
#14900=LINE ( 'NONE', #3553, #14914 ) ;
#14904=EDGE_CURVE ( 'NONE', #24509, #6270, #11181, .T. ) ;
#14907=ORIENTED_EDGE ( 'NONE', *, *, #1300, .T. ) ;
#14914=VECTOR ( 'NONE', #12856, 1000.000000000000114 ) ;
#14925=VERTEX_POINT ( 'NONE', #15418 ) ;
#14935=DIRECTION ( 'NONE',  ( 1.000000000000000000, 0.000000000000000000, -1.734723475976814737E-16 ) ) ;
#14966=CARTESIAN_POINT ( 'NONE',  ( 44.81606138205700063, 39.39281886181299797, 81.75501292736983316 ) ) ;
#14988=AXIS2_PLACEMENT_3D ( 'NONE', #24227, #20005, #24105 ) ;
#14993=ORIENTED_EDGE ( 'NONE', *, *, #17309, .F. ) ;
#14995=LINE ( 'NONE', #17067, #3267 ) ;
#15023=ORIENTED_EDGE ( 'NONE', *, *, #11687, .T. ) ;
#15047=LINE ( 'NONE', #23029, #835 ) ;
#15048=ORIENTED_EDGE ( 'NONE', *, *, #15465, .F. ) ;
#15060=EDGE_CURVE ( 'NONE', #21390, #14213, #16988, .T. ) ;
#15068=ADVANCED_FACE ( 'NONE', ( #16042 ), #571, .T. ) ;
#15082=ORIENTED_EDGE ( 'NONE', *, *, #15615, .F. ) ;
#15092=LINE ( 'NONE', #20513, #23970 ) ;
#15097=DIRECTION ( 'NONE',  ( -1.000000000000000000, 6.018531076210110289E-31, 1.734723475976804876E-16 ) ) ;
#15101=DIRECTION ( 'NONE',  ( -1.000000000000000000, 0.000000000000000000, 0.000000000000000000 ) ) ;
#15116=DIRECTION ( 'NONE',  ( -1.000000000000000000, -1.734723475976804876E-16, 1.734723475976814737E-16 ) ) ;
#15138=PLANE ( 'NONE',  #21103 ) ;
#15147=CARTESIAN_POINT ( 'NONE',  ( 30.81606138205700418, -26.74044063519535186, 82.55501292737007191 ) ) ;
#15179=PLANE ( 'NONE',  #20656 ) ;
#15214=LINE ( 'NONE', #13299, #20460 ) ;
#15221=CARTESIAN_POINT ( 'NONE',  ( 44.06606138205700063, 40.39281886181299797, 84.30501292736984453 ) ) ;
#15243=ORIENTED_EDGE ( 'NONE', *, *, #1686, .T. ) ;
#15245=DIRECTION ( 'NONE',  ( -6.489379976170840313E-31, 1.000000000000000000, -3.491481338843135327E-15 ) ) ;
#15271=DIRECTION ( 'NONE',  ( -1.734723475976804876E-16, -3.491481338843135327E-15, -1.000000000000000000 ) ) ;
#15275=CARTESIAN_POINT ( 'NONE',  ( 44.81606138205700063, -21.15876147765410309, 66.30501292737000085 ) ) ;
#15291=PLANE ( 'NONE',  #4005 ) ;
#15292=EDGE_CURVE ( 'NONE', #5806, #21711, #8841, .T. ) ;
#15301=ORIENTED_EDGE ( 'NONE', *, *, #10516, .T. ) ;
#15311=SHAPE_REPRESENTATION_RELATIONSHIP ( 'NONE' , 'NONE' ,  #14684, #15967 ) ;
#15312=ORIENTED_EDGE ( 'NONE', *, *, #7450, .F. ) ;
#15313=CARTESIAN_POINT ( 'NONE',  ( 30.81606138205700418, -34.55876147765410167, 66.30501292737000085 ) ) ;
#15316=ORIENTED_EDGE ( 'NONE', *, *, #4831, .T. ) ;
#15322=DIRECTION ( 'NONE',  ( 1.734723475976804876E-16, -1.000000000000000000, -3.009265538105065326E-32 ) ) ;
#15325=LINE ( 'NONE', #9543, #5513 ) ;
#15348=DIRECTION ( 'NONE',  ( -1.000000000000000000, 1.809068767804384992E-15, 0.000000000000000000 ) ) ;
#15372=CYLINDRICAL_SURFACE ( 'NONE', #10839, 1.000000000000000888 ) ;
#15377=AXIS2_PLACEMENT_3D ( 'NONE', #16292, #24022, #2883 ) ;
#15378=LINE ( 'NONE', #1961, #16563 ) ;
#15380=CARTESIAN_POINT ( 'NONE',  ( 30.81606138205700418, 40.39281886181299797, 81.75501292736983316 ) ) ;
#15385=EDGE_CURVE ( 'NONE', #18741, #131, #20675, .T. ) ;
#15387=APPLICATION_CONTEXT ( 'automotive_design' ) ;
#15415=ORIENTED_EDGE ( 'NONE', *, *, #4067, .F. ) ;
#15418=CARTESIAN_POINT ( 'NONE',  ( 41.32070064951228971, -37.35828293338759920, 84.30501292737011454 ) ) ;
#15419=DIRECTION ( 'NONE',  ( 0.000000000000000000, 1.000000000000000000, -3.469446951953614189E-15 ) ) ;
#15430=VECTOR ( 'NONE', #511, 1000.000000000000000 ) ;
#15442=DIRECTION ( 'NONE',  ( -1.000000000000000000, -6.505213034913019208E-17, 1.734723475976809806E-16 ) ) ;
#15465=EDGE_CURVE ( 'NONE', #21490, #22425, #15378, .T. ) ;
#15469=VERTEX_POINT ( 'NONE', #1838 ) ;
#15470=LINE ( 'NONE', #13546, #11752 ) ;
#15474=LINE ( 'NONE', #7887, #3764 ) ;
#15479=CARTESIAN_POINT ( 'NONE',  ( 30.81606138205700418, -26.74044063519544778, 66.30501292737000085 ) ) ;
#15509=DIRECTION ( 'NONE',  ( -1.000000000000000000, 6.018531076210110289E-31, 1.734723475976804876E-16 ) ) ;
#15515=ORIENTED_EDGE ( 'NONE', *, *, #10395, .F. ) ;
#15527=ADVANCED_FACE ( 'NONE', ( #9473 ), #25144, .F. ) ;
#15528=VECTOR ( 'NONE', #21038, 1000.000000000000000 ) ;
#15533=ORIENTED_EDGE ( 'NONE', *, *, #7097, .T. ) ;
#15538=EDGE_CURVE ( 'NONE', #1971, #3634, #9602, .T. ) ;
#15541=VERTEX_POINT ( 'NONE', #17451 ) ;
#15545=DIRECTION ( 'NONE',  ( -1.000000000000000000, 4.513898307157560384E-31, 1.734723475976809806E-16 ) ) ;
#15552=ORIENTED_EDGE ( 'NONE', *, *, #284, .T. ) ;
#15554=VERTEX_POINT ( 'NONE', #3776 ) ;
#15563=ORIENTED_EDGE ( 'NONE', *, *, #11969, .T. ) ;
#15610=AXIS2_PLACEMENT_3D ( 'NONE', #20951, #15271, #24908 ) ;
#15615=EDGE_CURVE ( 'NONE', #4487, #22083, #14121, .T. ) ;
#15642=ORIENTED_EDGE ( 'NONE', *, *, #14426, .F. ) ;
#15645=CARTESIAN_POINT ( 'NONE',  ( 30.81606138205700418, 40.39281886181299797, 84.30501292736984453 ) ) ;
#15647=AXIS2_PLACEMENT_3D ( 'NONE', #18704, #2839, #20507 ) ;
#15657=DIRECTION ( 'NONE',  ( 1.734723475976804876E-16, 3.269436733918100469E-15, 1.000000000000000000 ) ) ;
#15672=ORIENTED_EDGE ( 'NONE', *, *, #15707, .T. ) ;
#15681=LINE ( 'NONE', #23528, #21750 ) ;
#15685=DIRECTION ( 'NONE',  ( 1.734723475976804876E-16, 3.491481338843135327E-15, 1.000000000000000000 ) ) ;
#15686=ORIENTED_EDGE ( 'NONE', *, *, #7660, .F. ) ;
#15687=EDGE_LOOP ( 'NONE', ( #20543, #23299 ) ) ;
#15699=ORIENTED_EDGE ( 'NONE', *, *, #13511, .F. ) ;
#15700=CARTESIAN_POINT ( 'NONE',  ( 44.06606138205700063, -26.74044063519535186, 82.55501292737007191 ) ) ;
#15702=CARTESIAN_POINT ( 'NONE',  ( 31.81606138205700418, -34.55876147765410167, 70.30501292737000085 ) ) ;
#15707=EDGE_CURVE ( 'NONE', #19809, #3263, #11666, .T. ) ;
#15712=EDGE_CURVE ( 'NONE', #6422, #18550, #8291, .T. ) ;
#15716=ORIENTED_EDGE ( 'NONE', *, *, #4379, .F. ) ;
#15725=EDGE_CURVE ( 'NONE', #14027, #6661, #16379, .T. ) ;
#15749=VECTOR ( 'NONE', #3822, 1000.000000000000000 ) ;
#15772=DIRECTION ( 'NONE',  ( 4.336808689942074435E-17, -1.000000000000000000, 3.491481338843135327E-15 ) ) ;
#15777=( GEOMETRIC_REPRESENTATION_CONTEXT ( 3 ) GLOBAL_UNCERTAINTY_ASSIGNED_CONTEXT ( ( #20601 ) ) GLOBAL_UNIT_ASSIGNED_CONTEXT ( ( #21242, #25076, #11340 ) ) REPRESENTATION_CONTEXT ( 'NONE', 'WORKASPACE' ) );
#15783=PLANE ( 'NONE',  #25368 ) ;
#15786=ORIENTED_EDGE ( 'NONE', *, *, #6026, .F. ) ;
#15788=CARTESIAN_POINT ( 'NONE',  ( 41.14099152588522657, 1.392818861812999964, 83.30501292736997243 ) ) ;
#15802=FACE_OUTER_BOUND ( 'NONE', #1162, .T. ) ;
#15811=LINE ( 'NONE', #21738, #5692 ) ;
#15819=EDGE_LOOP ( 'NONE', ( #22604, #1292 ) ) ;
#15825=LINE ( 'NONE', #2162, #16147 ) ;
#15839=EDGE_LOOP ( 'NONE', ( #25425, #8288, #9533, #14378 ) ) ;
#15847=ADVANCED_FACE ( 'NONE', ( #12797 ), #18967, .F. ) ;
#15851=PLANE ( 'NONE',  #9674 ) ;
#15854=EDGE_CURVE ( 'NONE', #21433, #13492, #15092, .T. ) ;
#15862=EDGE_CURVE ( 'NONE', #24921, #7305, #13043, .T. ) ;
#15871=EDGE_CURVE ( 'NONE', #16610, #21433, #18579, .T. ) ;
#15876=LINE ( 'NONE', #4668, #11936 ) ;
#15889=ORIENTED_EDGE ( 'NONE', *, *, #13000, .F. ) ;
#15901=DIRECTION ( 'NONE',  ( 1.734723475976814737E-16, -1.000000000000000000, 3.491481338843135327E-15 ) ) ;
#15920=CARTESIAN_POINT ( 'NONE',  ( 31.81606138205700418, -34.67340937580780036, 71.26505871168839690 ) ) ;
#15928=CYLINDRICAL_SURFACE ( 'NONE', #18485, 12.59999999999999964 ) ;
#15931=PLANE ( 'NONE',  #18095 ) ;
#15935=AXIS2_PLACEMENT_3D ( 'NONE', #7701, #15545, #23394 ) ;
#15936=EDGE_CURVE ( 'NONE', #12560, #24557, #20899, .T. ) ;
#15937=PLANE ( 'NONE',  #20602 ) ;
#15942=PLANE ( 'NONE',  #21484 ) ;
#15967=ADVANCED_BREP_SHAPE_REPRESENTATION ( '', ( #16726, #2000 ), #15777 ) ;
#15971=DIRECTION ( 'NONE',  ( 1.734723475976804876E-16, 3.491481338843135327E-15, 1.000000000000000000 ) ) ;
#15974=DIRECTION ( 'NONE',  ( 1.734723475976814737E-16, -1.000000000000000000, 3.491481338843135327E-15 ) ) ;
#15976=LINE ( 'NONE', #2446, #15430 ) ;
#16003=ORIENTED_EDGE ( 'NONE', *, *, #19763, .F. ) ;
#16006=EDGE_CURVE ( 'NONE', #21390, #15554, #17546, .T. ) ;
#16012=ORIENTED_EDGE ( 'NONE', *, *, #19494, .T. ) ;
#16022=EDGE_CURVE ( 'NONE', #20938, #18511, #21124, .T. ) ;
#16039=VERTEX_POINT ( 'NONE', #3881 ) ;
#16042=FACE_OUTER_BOUND ( 'NONE', #19231, .T. ) ;
#16051=EDGE_LOOP ( 'NONE', ( #6510, #21581, #18364, #4319 ) ) ;
#16065=ORIENTED_EDGE ( 'NONE', *, *, #17309, .T. ) ;
#16071=FACE_OUTER_BOUND ( 'NONE', #1154, .T. ) ;
#16073=AXIS2_PLACEMENT_3D ( 'NONE', #13473, #13234, #1726 ) ;
#16077=EDGE_CURVE ( 'NONE', #18272, #15541, #10025, .T. ) ;
#16099=DIRECTION ( 'NONE',  ( 1.000000000000000000, 0.000000000000000000, 0.000000000000000000 ) ) ;
#16111=CARTESIAN_POINT ( 'NONE',  ( 40.64099152588523367, 1.392818861812999964, 93.30501292736998664 ) ) ;
#16117=VECTOR ( 'NONE', #21340, 1000.000000000000000 ) ;
#16134=LINE ( 'NONE', #8293, #989 ) ;
#16145=CARTESIAN_POINT ( 'NONE',  ( 44.81606138205700063, -38.55876147765410167, 70.30501292737011454 ) ) ;
#16147=VECTOR ( 'NONE', #10417, 1000.000000000000000 ) ;
#16164=AXIS2_PLACEMENT_3D ( 'NONE', #2845, #1306, #4792 ) ;
#16165=CARTESIAN_POINT ( 'NONE',  ( 44.06606138205700063, 40.39281886181299797, 82.55501292736983032 ) ) ;
#16174=ADVANCED_FACE ( 'NONE', ( #4519 ), #4144, .F. ) ;
#16187=VECTOR ( 'NONE', #21028, 1000.000000000000000 ) ;
#16189=ADVANCED_FACE ( 'NONE', ( #20101 ), #6569, .F. ) ;
#16200=CIRCLE ( 'NONE', #5108, 3.000000000000002665 ) ;
#16211=VECTOR ( 'NONE', #13706, 1000.000000000000000 ) ;
#16221=EDGE_LOOP ( 'NONE', ( #3923, #3733, #4327, #1759 ) ) ;
#16249=CARTESIAN_POINT ( 'NONE',  ( 45.81606138205700063, 40.39281886181299797, 80.75501292736983316 ) ) ;
#16258=ORIENTED_EDGE ( 'NONE', *, *, #19326, .F. ) ;
#16285=ORIENTED_EDGE ( 'NONE', *, *, #22486, .F. ) ;
#16292=CARTESIAN_POINT ( 'NONE',  ( 44.06606138205700063, 43.35512946304240245, 83.12823623207320622 ) ) ;
#16295=ORIENTED_EDGE ( 'NONE', *, *, #18172, .F. ) ;
#16325=AXIS2_PLACEMENT_3D ( 'NONE', #23075, #17168, #6991 ) ;
#16327=LINE ( 'NONE', #4623, #23947 ) ;
#16328=AXIS2_PLACEMENT_3D ( 'NONE', #1591, #17329, #25154 ) ;
#16348=CARTESIAN_POINT ( 'NONE',  ( 32.56606138205700773, -26.74044063519535186, 82.55501292737007191 ) ) ;
#16352=DIRECTION ( 'NONE',  ( -1.734723475976804876E-16, -3.469446951953610245E-15, -1.000000000000000000 ) ) ;
#16358=ADVANCED_FACE ( 'NONE', ( #24452 ), #24707, .F. ) ;
#16368=CARTESIAN_POINT ( 'NONE',  ( 44.81606138205700063, 40.39281886181299797, 81.75501292736983316 ) ) ;
#16379=LINE ( 'NONE', #24228, #928 ) ;
#16384=CARTESIAN_POINT ( 'NONE',  ( 32.56606138205700773, 40.39281886181299797, 83.30501292736984453 ) ) ;
#16390=ADVANCED_FACE ( 'NONE', ( #24572 ), #6693, .F. ) ;
#16391=FACE_OUTER_BOUND ( 'NONE', #12550, .T. ) ;
#16402=EDGE_LOOP ( 'NONE', ( #18576, #24295, #8832, #22944 ) ) ;
#16420=VECTOR ( 'NONE', #3189, 1000.000000000000000 ) ;
#16425=ORIENTED_EDGE ( 'NONE', *, *, #19494, .F. ) ;
#16437=AXIS2_PLACEMENT_3D ( 'NONE', #19853, #5686, #19341 ) ;
#16438=PLANE ( 'NONE',  #22238 ) ;
#16440=VERTEX_POINT ( 'NONE', #4642 ) ;
#16443=VECTOR ( 'NONE', #24695, 1000.000000000000000 ) ;
#16447=DIRECTION ( 'NONE',  ( 1.000000000000000000, 1.734723475976804876E-16, -1.734723475976814737E-16 ) ) ;
#16450=CIRCLE ( 'NONE', #17698, 2.000000000000001776 ) ;
#16463=ADVANCED_FACE ( 'NONE', ( #12522 ), #7855, .F. ) ;
#16494=DIRECTION ( 'NONE',  ( -1.734723475976804876E-16, 1.000000000000000000, 0.000000000000000000 ) ) ;
#16530=ORIENTED_EDGE ( 'NONE', *, *, #21999, .T. ) ;
#16533=ORIENTED_EDGE ( 'NONE', *, *, #9081, .F. ) ;
#16538=EDGE_LOOP ( 'NONE', ( #12819, #9739, #913, #5594 ) ) ;
#16548=AXIS2_PLACEMENT_3D ( 'NONE', #13863, #11947, #5751 ) ;
#16563=VECTOR ( 'NONE', #11400, 1000.000000000000000 ) ;
#16582=VECTOR ( 'NONE', #7130, 1000.000000000000000 ) ;
#16585=CARTESIAN_POINT ( 'NONE',  ( 15.14989484155900001, 36.04731275961434989, 83.30501292736985874 ) ) ;
#16591=AXIS2_PLACEMENT_3D ( 'NONE', #22578, #22328, #10871 ) ;
#16594=VERTEX_POINT ( 'NONE', #5785 ) ;
#16607=DIRECTION ( 'NONE',  ( 1.000000000000000000, 6.071532165918830747E-16, -1.734723475976829774E-16 ) ) ;
#16610=VERTEX_POINT ( 'NONE', #13644 ) ;
#16634=ORIENTED_EDGE ( 'NONE', *, *, #15292, .F. ) ;
#16655=EDGE_CURVE ( 'NONE', #17608, #5806, #10868, .T. ) ;
#16657=DIRECTION ( 'NONE',  ( -1.000000000000000000, -1.734723475976804876E-16, 1.734723475976814737E-16 ) ) ;
#16662=CARTESIAN_POINT ( 'NONE',  ( 31.81606138205700418, -21.15876147765410309, 66.30501292737000085 ) ) ;
#16672=PLANE ( 'NONE',  #10289 ) ;
#16678=ORIENTED_EDGE ( 'NONE', *, *, #7053, .T. ) ;
#16684=AXIS2_PLACEMENT_3D ( 'NONE', #16348, #18308, #16099 ) ;
#16726=MANIFOLD_SOLID_BREP ( 'NONE', #14693 ) ;
#16761=VERTEX_POINT ( 'NONE', #6772 ) ;
#16778=EDGE_LOOP ( 'NONE', ( #528, #10785, #24289, #17148 ) ) ;
#16780=VECTOR ( 'NONE', #23782, 1000.000000000000000 ) ;
#16806=CARTESIAN_POINT ( 'NONE',  ( 44.06606138205700063, 47.04446929126260102, 81.37823623207319201 ) ) ;
#16812=VERTEX_POINT ( 'NONE', #3408 ) ;
#16820=DIRECTION ( 'NONE',  ( 1.000000000000000000, 2.168404344971010101E-16, -1.734723475976814737E-16 ) ) ;
#16827=DIRECTION ( 'NONE',  ( 1.000000000000000000, 1.734723475976799945E-16, -1.734723475976814737E-16 ) ) ;
#16852=LINE ( 'NONE', #20459, #22934 ) ;
#16856=DIRECTION ( 'NONE',  ( -1.734723475976814737E-16, 1.000000000000000000, -3.491481338843135327E-15 ) ) ;
#16863=ORIENTED_EDGE ( 'NONE', *, *, #8448, .T. ) ;
#16864=ORIENTED_EDGE ( 'NONE', *, *, #13806, .T. ) ;
#16876=DIRECTION ( 'NONE',  ( 5.047295537021760406E-31, -1.000000000000000000, 3.491481338843135327E-15 ) ) ;
#16887=AXIS2_PLACEMENT_3D ( 'NONE', #10811, #2931, #7205 ) ;
#16890=ORIENTED_EDGE ( 'NONE', *, *, #7183, .F. ) ;
#16898=ORIENTED_EDGE ( 'NONE', *, *, #1627, .T. ) ;
#16904=CIRCLE ( 'NONE', #23066, 4.000000000000000000 ) ;
#16914=FACE_OUTER_BOUND ( 'NONE', #14692, .T. ) ;
#16922=CARTESIAN_POINT ( 'NONE',  ( 32.56606138205700773, 43.35512946304240245, 83.12823623207320622 ) ) ;
#16925=AXIS2_PLACEMENT_3D ( 'NONE', #7570, #25438, #15419 ) ;
#16944=AXIS2_PLACEMENT_3D ( 'NONE', #22124, #10287, #18278 ) ;
#16947=CARTESIAN_POINT ( 'NONE',  ( 35.64099152588523367, -8.607181138186998481, 93.30501292736998664 ) ) ;
#16957=AXIS2_PLACEMENT_3D ( 'NONE', #22640, #4993, #11321 ) ;
#16962=CARTESIAN_POINT ( 'NONE',  ( 41.32070064951228971, -37.35828293338759920, 83.30501292737011454 ) ) ;
#16967=ORIENTED_EDGE ( 'NONE', *, *, #24479, .F. ) ;
#16971=ORIENTED_EDGE ( 'NONE', *, *, #7604, .T. ) ;
#16985=CARTESIAN_POINT ( 'NONE',  ( 32.56606138205700773, 42.11769259596595560, 81.89079936499673806 ) ) ;
#16988=CIRCLE ( 'NONE', #16548, 0.7500000000000006661 ) ;
#16990=CARTESIAN_POINT ( 'NONE',  ( 38.31606138205699352, 47.04446929126260102, 82.37823623207320622 ) ) ;
#16991=EDGE_CURVE ( 'NONE', #23473, #22425, #11537, .T. ) ;
#16993=FACE_OUTER_BOUND ( 'NONE', #17081, .T. ) ;
#17011=DIRECTION ( 'NONE',  ( -1.734723475976814737E-16, 1.000000000000000000, -3.491481338843135327E-15 ) ) ;
#17014=STYLED_ITEM ( 'NONE', ( #7461 ), #15967 ) ;
#17020=VERTEX_POINT ( 'NONE', #17456 ) ;
#17029=ORIENTED_EDGE ( 'NONE', *, *, #15854, .F. ) ;
#17045=MECHANICAL_DESIGN_GEOMETRIC_PRESENTATION_REPRESENTATION('',(#4700),#24004);
#17047=ORIENTED_EDGE ( 'NONE', *, *, #13211, .T. ) ;
#17057=PRODUCT_DEFINITION_FORMATION_WITH_SPECIFIED_SOURCE ( 'ANY', '', #9935, .NOT_KNOWN. ) ;
#17059=EDGE_CURVE ( 'NONE', #14925, #13947, #25406, .T. ) ;
#17064=VERTEX_POINT ( 'NONE', #8548 ) ;
#17066=ORIENTED_EDGE ( 'NONE', *, *, #16655, .F. ) ;
#17067=CARTESIAN_POINT ( 'NONE',  ( 31.81606138205700418, -26.97987052895604876, 80.55501292737007191 ) ) ;
#17068=DIRECTION ( 'NONE',  ( 0.000000000000000000, 1.000000000000000000, 0.000000000000000000 ) ) ;
#17081=EDGE_LOOP ( 'NONE', ( #6979, #3430, #41, #13261 ) ) ;
#17082=ORIENTED_EDGE ( 'NONE', *, *, #13429, .T. ) ;
#17083=CARTESIAN_POINT ( 'NONE',  ( 31.81606138205700418, -30.95005513552129983, 81.04249030099066431 ) ) ;
#17091=CARTESIAN_POINT ( 'NONE',  ( 30.81606138205700418, 40.39281886181299797, 66.30501292737000085 ) ) ;
#17096=ORIENTED_EDGE ( 'NONE', *, *, #7196, .T. ) ;
#17108=CARTESIAN_POINT ( 'NONE',  ( 40.64099152588522657, -9.607181138187000258, 80.05501292737000085 ) ) ;
#17117=DIRECTION ( 'NONE',  ( 5.047295537021760406E-31, -1.000000000000000000, 3.491481338843135327E-15 ) ) ;
#17119=LINE ( 'NONE', #19415, #5327 ) ;
#17120=EDGE_CURVE ( 'NONE', #7648, #7039, #16134, .T. ) ;
#17136=LINE ( 'NONE', #7342, #20540 ) ;
#17146=CARTESIAN_POINT ( 'NONE',  ( 31.81606138205700418, -3.831401139557048197, 80.75501292737000369 ) ) ;
#17148=ORIENTED_EDGE ( 'NONE', *, *, #6149, .F. ) ;
#17168=DIRECTION ( 'NONE',  ( -1.000000000000000000, -1.950367120401949903E-17, 2.478176394252580155E-16 ) ) ;
#17183=VERTEX_POINT ( 'NONE', #14589 ) ;
#17186=DIRECTION ( 'NONE',  ( -1.000000000000000000, -2.156013462999745228E-15, 0.000000000000000000 ) ) ;
#17187=CARTESIAN_POINT ( 'NONE',  ( 32.56606138205700773, -26.74044063519535186, 82.55501292737007191 ) ) ;
#17189=ORIENTED_EDGE ( 'NONE', *, *, #9290, .T. ) ;
#17191=CARTESIAN_POINT ( 'NONE',  ( 31.81606138205700418, -26.74044063519535186, 82.50501292737007475 ) ) ;
#17203=ORIENTED_EDGE ( 'NONE', *, *, #19452, .T. ) ;
#17219=DIRECTION ( 'NONE',  ( 1.734723475976814737E-16, -1.000000000000000000, 3.491481338843135327E-15 ) ) ;
#17222=DIRECTION ( 'NONE',  ( -1.000000000000000000, 6.018531076210110289E-31, 1.734723475976804876E-16 ) ) ;
#17227=CYLINDRICAL_SURFACE ( 'NONE', #14096, 1.750000000000001554 ) ;
#17234=DIRECTION ( 'NONE',  ( 1.734723475976814737E-16, -1.000000000000000000, 3.491481338843135327E-15 ) ) ;
#17244=LINE ( 'NONE', #21234, #2872 ) ;
#17264=LINE ( 'NONE', #5415, #23175 ) ;
#17265=CIRCLE ( 'NONE', #11527, 10.00000000000000000 ) ;
#17269=AXIS2_PLACEMENT_3D ( 'NONE', #18203, #4548, #4418 ) ;
#17283=DIRECTION ( 'NONE',  ( 1.734723475976814737E-16, -1.000000000000000000, 3.491481338843135327E-15 ) ) ;
#17293=DIRECTION ( 'NONE',  ( 1.734723475976814737E-16, -1.000000000000000000, 3.491481338843135327E-15 ) ) ;
#17297=DIRECTION ( 'NONE',  ( -1.000000000000000000, 6.018531076210110289E-31, 1.734723475976804876E-16 ) ) ;
#17309=EDGE_CURVE ( 'NONE', #24921, #22752, #15474, .T. ) ;
#17318=ORIENTED_EDGE ( 'NONE', *, *, #23339, .T. ) ;
#17329=DIRECTION ( 'NONE',  ( -1.734723475976814737E-16, 1.000000000000000000, -3.491481338843135327E-15 ) ) ;
#17337=DIRECTION ( 'NONE',  ( -0.000000000000000000, 1.000000000000000000, 0.000000000000000000 ) ) ;
#17340=VERTEX_POINT ( 'NONE', #21276 ) ;
#17348=VERTEX_POINT ( 'NONE', #1552 ) ;
#17363=CARTESIAN_POINT ( 'NONE',  ( 44.81606138205700063, -26.97987052895604876, 80.55501292737007191 ) ) ;
#17378=FILL_AREA_STYLE_COLOUR ( '', #21130 ) ;
#17407=DIRECTION ( 'NONE',  ( -2.453269466693404537E-16, 0.7071067811865489050, -0.7071067811865460184 ) ) ;
#17414=CARTESIAN_POINT ( 'NONE',  ( 44.06606138205700063, 40.39281886181299797, 83.30501292736984453 ) ) ;
#17422=AXIS2_PLACEMENT_3D ( 'NONE', #25000, #23208, #23081 ) ;
#17443=FACE_OUTER_BOUND ( 'NONE', #13417, .T. ) ;
#17450=COLOUR_RGB ( '', 0.40784314, 0.44705882, 0.49803922) ;
#17451=CARTESIAN_POINT ( 'NONE',  ( 32.56606138205700773, 42.82479937715250173, 82.59790614618330551 ) ) ;
#17456=CARTESIAN_POINT ( 'NONE',  ( 45.81606138205700063, -26.74044063519535186, 82.55501292737007191 ) ) ;
#17459=ORIENTED_EDGE ( 'NONE', *, *, #7450, .T. ) ;
#17475=ADVANCED_FACE ( 'NONE', ( #10195 ), #8395, .T. ) ;
#17492=VECTOR ( 'NONE', #660, 1000.000000000000000 ) ;
#17496=LINE ( 'NONE', #3560, #15749 ) ;
#17505=DIRECTION ( 'NONE',  ( 1.000000000000000000, -6.018531076210090146E-31, -1.734723475976804876E-16 ) ) ;
#17530=ORIENTED_EDGE ( 'NONE', *, *, #10395, .T. ) ;
#17538=PRODUCT_DEFINITION_SHAPE ( 'NONE', 'NONE',  #3162 ) ;
#17540=VERTEX_POINT ( 'NONE', #2948 ) ;
#17546=LINE ( 'NONE', #17414, #5916 ) ;
#17567=CARTESIAN_POINT ( 'NONE',  ( 44.06606138205700063, -26.74044063519535186, 84.30501292737007191 ) ) ;
#17572=CARTESIAN_POINT ( 'NONE',  ( 35.64099152588522657, -8.607181138186998481, 83.30501292737001506 ) ) ;
#17585=DIRECTION ( 'NONE',  ( 0.000000000000000000, 1.000000000000000000, -3.469446951953701358E-15 ) ) ;
#17601=AXIS2_PLACEMENT_3D ( 'NONE', #18589, #10872, #15101 ) ;
#17608=VERTEX_POINT ( 'NONE', #11086 ) ;
#17651=DIRECTION ( 'NONE',  ( 1.000000000000000000, 1.734723475976804876E-16, -1.734723475976814737E-16 ) ) ;
#17660=ADVANCED_FACE ( 'NONE', ( #14677 ), #22545, .F. ) ;
#17678=DIRECTION ( 'NONE',  ( 0.000000000000000000, -0.7071067811865489050, 0.7071067811865460184 ) ) ;
#17686=EDGE_CURVE ( 'NONE', #4783, #7140, #13676, .T. ) ;
#17695=CARTESIAN_POINT ( 'NONE',  ( 38.38987944808049235, -39.60718113818700203, 83.30501292737011454 ) ) ;
#17696=CARTESIAN_POINT ( 'NONE',  ( 31.81606138205700418, -36.05876147765410877, 70.30501292737000085 ) ) ;
#17698=AXIS2_PLACEMENT_3D ( 'NONE', #257, #8136, #22804 ) ;
#17717=DIRECTION ( 'NONE',  ( 0.000000000000000000, -4.343580702399009298E-14, -1.000000000000000000 ) ) ;
#17719=DIRECTION ( 'NONE',  ( -1.000000000000000000, -1.734723475976804876E-16, 1.734723475976814737E-16 ) ) ;
#17720=VECTOR ( 'NONE', #12127, 1000.000000000000000 ) ;
#17744=VECTOR ( 'NONE', #21325, 1000.000000000000000 ) ;
#17748=FACE_OUTER_BOUND ( 'NONE', #12411, .T. ) ;
#17750=FACE_OUTER_BOUND ( 'NONE', #8643, .T. ) ;
#17751=CARTESIAN_POINT ( 'NONE',  ( 17.31606138205699708, 34.87886987267149408, 81.44836866983821722 ) ) ;
#17760=ORIENTED_EDGE ( 'NONE', *, *, #9883, .T. ) ;
#17761=CIRCLE ( 'NONE', #16925, 4.000000000000000000 ) ;
#17766=AXIS2_PLACEMENT_3D ( 'NONE', #12145, #19984, #508 ) ;
#17800=ORIENTED_EDGE ( 'NONE', *, *, #16655, .T. ) ;
#17822=AXIS2_PLACEMENT_3D ( 'NONE', #5255, #24548, #856 ) ;
#17831=ORIENTED_EDGE ( 'NONE', *, *, #11009, .F. ) ;
#17839=CARTESIAN_POINT ( 'NONE',  ( 31.81606138205700418, -38.55876147765429351, 66.30501292737328356 ) ) ;
#17845=DIRECTION ( 'NONE',  ( 1.000000000000000000, 2.168404344971055214E-16, -1.734723475976814737E-16 ) ) ;
#17846=AXIS2_PLACEMENT_3D ( 'NONE', #8818, #16657, #3121 ) ;
#17852=CIRCLE ( 'NONE', #3859, 10.00000000000000000 ) ;
#17856=CARTESIAN_POINT ( 'NONE',  ( 44.81606138205700063, 40.39281886181299797, 66.30501292737000085 ) ) ;
#17875=CARTESIAN_POINT ( 'NONE',  ( 34.56606138205700773, 47.04446929126254417, 81.37823623207319201 ) ) ;
#17877=EDGE_LOOP ( 'NONE', ( #2555, #829, #10859, #7485 ) ) ;
#17880=CARTESIAN_POINT ( 'NONE',  ( 45.81606138205700063, -21.15876147765410309, 66.30501292737000085 ) ) ;
#17888=CARTESIAN_POINT ( 'NONE',  ( 45.81606138205700063, -38.55876147765399509, 84.30501292737011454 ) ) ;
#17893=LINE ( 'NONE', #217, #19346 ) ;
#17895=ORIENTED_EDGE ( 'NONE', *, *, #13344, .T. ) ;
#17908=VECTOR ( 'NONE', #22059, 1000.000000000000000 ) ;
#17914=CARTESIAN_POINT ( 'NONE',  ( 40.64099152588522657, 0.3928188618129990761, 83.02501292736999972 ) ) ;
#17938=EDGE_CURVE ( 'NONE', #3263, #14925, #3038, .T. ) ;
#17940=EDGE_CURVE ( 'NONE', #21036, #6661, #22304, .T. ) ;
#17942=DIRECTION ( 'NONE',  ( -1.734723475976804876E-16, 1.000000000000000000, 3.009265538105065326E-32 ) ) ;
#17984=EDGE_CURVE ( 'NONE', #2290, #3395, #8988, .T. ) ;
#17994=CARTESIAN_POINT ( 'NONE',  ( 41.14099152588522657, -10.60718113818700026, 83.30501292737001506 ) ) ;
#17998=VECTOR ( 'NONE', #24500, 1000.000000000000000 ) ;
#18011=CARTESIAN_POINT ( 'NONE',  ( 45.81606138205700063, -36.05876147765410877, 70.30501292737000085 ) ) ;
#18023=ORIENTED_EDGE ( 'NONE', *, *, #24650, .T. ) ;
#18024=DIRECTION ( 'NONE',  ( -1.734723475976814737E-16, 1.000000000000000000, -3.491481338843135327E-15 ) ) ;
#18036=CARTESIAN_POINT ( 'NONE',  ( 44.81606138205700063, 40.39281886181299797, 84.30501292736984453 ) ) ;
#18087=VERTEX_POINT ( 'NONE', #15788 ) ;
#18094=EDGE_CURVE ( 'NONE', #13492, #22911, #23644, .T. ) ;
#18095=AXIS2_PLACEMENT_3D ( 'NONE', #10276, #334, #8346 ) ;
#18097=VECTOR ( 'NONE', #10798, 1000.000000000000000 ) ;
#18136=CARTESIAN_POINT ( 'NONE',  ( 35.64099152588523367, -0.6071811381869983704, 122.0250129273699997 ) ) ;
#18141=CARTESIAN_POINT ( 'NONE',  ( 44.06606138205700063, 40.39281886181299797, 84.30501292736984453 ) ) ;
#18145=DIRECTION ( 'NONE',  ( 0.000000000000000000, 1.000000000000000000, 0.000000000000000000 ) ) ;
#18149=DIRECTION ( 'NONE',  ( 1.734723475976814737E-16, 0.000000000000000000, 1.000000000000000000 ) ) ;
#18162=VECTOR ( 'NONE', #8076, 1000.000000000000000 ) ;
#18167=CARTESIAN_POINT ( 'NONE',  ( 30.81606138205700418, -33.05876147765410167, 70.30501292737000085 ) ) ;
#18172=EDGE_CURVE ( 'NONE', #4506, #4432, #16852, .T. ) ;
#18176=DIRECTION ( 'NONE',  ( 1.000000000000000000, 6.505213034913019208E-17, -1.734723475976809806E-16 ) ) ;
#18197=EDGE_CURVE ( 'NONE', #17183, #21390, #5138, .T. ) ;
#18203=CARTESIAN_POINT ( 'NONE',  ( 31.81606138205700418, 0.1601050959395486362, 68.80395113470939350 ) ) ;
#18232=ADVANCED_FACE ( 'NONE', ( #22263 ), #24434, .F. ) ;
#18233=CIRCLE ( 'NONE', #8784, 1.500000000000001332 ) ;
#18260=EDGE_CURVE ( 'NONE', #24890, #17540, #9792, .T. ) ;
#18266=FACE_OUTER_BOUND ( 'NONE', #21264, .T. ) ;
#18269=EDGE_CURVE ( 'NONE', #18272, #9258, #20846, .T. ) ;
#18272=VERTEX_POINT ( 'NONE', #10553 ) ;
#18278=DIRECTION ( 'NONE',  ( 0.000000000000000000, 1.000000000000000000, 0.000000000000000000 ) ) ;
#18280=VECTOR ( 'NONE', #22016, 1000.000000000000000 ) ;
#18287=CARTESIAN_POINT ( 'NONE',  ( 38.41621794735363693, -35.10729675983900222, 83.30501292737010033 ) ) ;
#18292=LINE ( 'NONE', #24528, #24028 ) ;
#18299=ORIENTED_EDGE ( 'NONE', *, *, #23741, .T. ) ;
#18308=DIRECTION ( 'NONE',  ( -5.047295537021760406E-31, 1.000000000000000000, -3.491481338843135327E-15 ) ) ;
#18334=ORIENTED_EDGE ( 'NONE', *, *, #12729, .T. ) ;
#18341=DIRECTION ( 'NONE',  ( 1.734723475976804876E-16, 3.491481338843135327E-15, 1.000000000000000000 ) ) ;
#18353=CARTESIAN_POINT ( 'NONE',  ( 44.06606138205700063, 40.39281886181299797, 84.30501292736984453 ) ) ;
#18364=ORIENTED_EDGE ( 'NONE', *, *, #19571, .T. ) ;
#18368=PRESENTATION_STYLE_ASSIGNMENT (( #20421 ) ) ;
#18373=CARTESIAN_POINT ( 'NONE',  ( 44.81606138205700063, -38.55876147765410167, 70.30501292737011454 ) ) ;
#18380=LINE ( 'NONE', #4603, #13898 ) ;
#18403=DIRECTION ( 'NONE',  ( -1.734723475976804876E-16, -3.491481338843135327E-15, -1.000000000000000000 ) ) ;
#18414=ORIENTED_EDGE ( 'NONE', *, *, #14602, .F. ) ;
#18417=ORIENTED_EDGE ( 'NONE', *, *, #14230, .F. ) ;
#18422=VECTOR ( 'NONE', #6609, 1000.000000000000114 ) ;
#18443=DIRECTION ( 'NONE',  ( -1.000000000000000000, -1.734723475976804876E-16, 1.734723475976814737E-16 ) ) ;
#18455=EDGE_LOOP ( 'NONE', ( #6288, #14322, #9592, #25310 ) ) ;
#18459=DIRECTION ( 'NONE',  ( -1.734723475976814737E-16, 1.000000000000000000, -3.491481338843135327E-15 ) ) ;
#18466=FACE_OUTER_BOUND ( 'NONE', #19372, .T. ) ;
#18474=LINE ( 'NONE', #14603, #5364 ) ;
#18485=AXIS2_PLACEMENT_3D ( 'NONE', #22110, #4350, #2269 ) ;
#18487=VERTEX_POINT ( 'NONE', #11707 ) ;
#18490=ADVANCED_FACE ( 'NONE', ( #13251 ), #15291, .T. ) ;
#18500=DIRECTION ( 'NONE',  ( 1.734723475976804876E-16, 3.252606517456515274E-15, 1.000000000000000000 ) ) ;
#18511=VERTEX_POINT ( 'NONE', #7444 ) ;
#18522=DIRECTION ( 'NONE',  ( -1.000000000000000000, -1.734723475976804876E-16, 1.734723475976814737E-16 ) ) ;
#18528=CARTESIAN_POINT ( 'NONE',  ( 44.81606138205700063, -34.55876147765410167, 66.30501292737000085 ) ) ;
#18532=EDGE_CURVE ( 'NONE', #9258, #11322, #6067, .T. ) ;
#18533=EDGE_CURVE ( 'NONE', #20770, #15469, #2354, .T. ) ;
#18534=CARTESIAN_POINT ( 'NONE',  ( 44.81606138205700063, -26.74044063519535186, 84.30501292737007191 ) ) ;
#18535=EDGE_CURVE ( 'NONE', #17183, #11291, #3591, .T. ) ;
#18550=VERTEX_POINT ( 'NONE', #12085 ) ;
#18558=CARTESIAN_POINT ( 'NONE',  ( 30.81606138205700418, 40.39281886181299797, 82.55501292736983032 ) ) ;
#18576=ORIENTED_EDGE ( 'NONE', *, *, #9414, .T. ) ;
#18579=LINE ( 'NONE', #8806, #5091 ) ;
#18585=ADVANCED_FACE ( 'NONE', ( #17748 ), #6021, .T. ) ;
#18586=CARTESIAN_POINT ( 'NONE',  ( 44.81606138205700063, -38.55876147765349771, 84.30501292737325514 ) ) ;
#18589=CARTESIAN_POINT ( 'NONE',  ( 32.56606138205700773, 40.39281886181299797, 82.55501292736983032 ) ) ;
#18592=LINE ( 'NONE', #8937, #5084 ) ;
#18593=DIRECTION ( 'NONE',  ( -1.734723475976804876E-16, -3.491481338843135327E-15, -1.000000000000000000 ) ) ;
#18616=EDGE_CURVE ( 'NONE', #6360, #10501, #8209, .T. ) ;
#18667=VECTOR ( 'NONE', #4375, 1000.000000000000000 ) ;
#18676=ORIENTED_EDGE ( 'NONE', *, *, #24453, .F. ) ;
#18701=ORIENTED_EDGE ( 'NONE', *, *, #8810, .T. ) ;
#18704=CARTESIAN_POINT ( 'NONE',  ( 32.56606138205700773, 43.35512946304240245, 83.12823623207320622 ) ) ;
#18706=EDGE_CURVE ( 'NONE', #13535, #19200, #9896, .T. ) ;
#18709=ORIENTED_EDGE ( 'NONE', *, *, #18172, .T. ) ;
#18710=DIRECTION ( 'NONE',  ( 1.000000000000000000, -6.018531076210080512E-31, -1.734723475976804876E-16 ) ) ;
#18719=PLANE ( 'NONE',  #21180 ) ;
#18721=ORIENTED_EDGE ( 'NONE', *, *, #18260, .F. ) ;
#18727=CYLINDRICAL_SURFACE ( 'NONE', #3423, 0.7500000000000006661 ) ;
#18735=ORIENTED_EDGE ( 'NONE', *, *, #1219, .T. ) ;
#18736=CARTESIAN_POINT ( 'NONE',  ( 41.14099152588522657, 1.392818861812999964, 84.30501292737000085 ) ) ;
#18741=VERTEX_POINT ( 'NONE', #22615 ) ;
#18768=CARTESIAN_POINT ( 'NONE',  ( 44.81606138205700063, 40.39281886181299797, 81.75501292736983316 ) ) ;
#18775=LINE ( 'NONE', #10676, #14071 ) ;
#18792=EDGE_LOOP ( 'NONE', ( #24366, #4311, #22977, #17800 ) ) ;
#18797=DIRECTION ( 'NONE',  ( 0.000000000000000000, -1.000000000000000000, 2.775557561562890957E-15 ) ) ;
#18810=CARTESIAN_POINT ( 'NONE',  ( 31.81606138205700418, 40.34464305740947054, 81.44836866983821722 ) ) ;
#18817=ORIENTED_EDGE ( 'NONE', *, *, #2787, .F. ) ;
#18840=VECTOR ( 'NONE', #5017, 1000.000000000000000 ) ;
#18842=VECTOR ( 'NONE', #6106, 1000.000000000000000 ) ;
#18853=EDGE_CURVE ( 'NONE', #18511, #21676, #12596, .T. ) ;
#18864=VECTOR ( 'NONE', #14881, 1000.000000000000000 ) ;
#18871=PLANE ( 'NONE',  #12415 ) ;
#18877=ORIENTED_EDGE ( 'NONE', *, *, #3899, .T. ) ;
#18880=LINE ( 'NONE', #4722, #7134 ) ;
#18882=ADVANCED_FACE ( 'NONE', ( #1088 ), #8975, .T. ) ;
#18889=DIRECTION ( 'NONE',  ( 0.000000000000000000, -1.000000000000000000, 2.775557561562890957E-15 ) ) ;
#18894=VERTEX_POINT ( 'NONE', #5107 ) ;
#18897=AXIS2_PLACEMENT_3D ( 'NONE', #21231, #17505, #23025 ) ;
#18908=VECTOR ( 'NONE', #16856, 1000.000000000000000 ) ;
#18910=ORIENTED_EDGE ( 'NONE', *, *, #8465, .F. ) ;
#18922=EDGE_LOOP ( 'NONE', ( #21835, #338, #25267, #14268 ) ) ;
#18936=DIRECTION ( 'NONE',  ( -1.000000000000000000, 0.000000000000000000, 0.000000000000000000 ) ) ;
#18944=CARTESIAN_POINT ( 'NONE',  ( 38.38987944808049235, -39.60718113818700203, 83.30501292737011454 ) ) ;
#18967=CYLINDRICAL_SURFACE ( 'NONE', #16164, 1.500000000000001332 ) ;
#18973=FACE_BOUND ( 'NONE', #21832, .T. ) ;
#18995=EDGE_LOOP ( 'NONE', ( #12419, #7014, #10380, #10826 ) ) ;
#19006=VECTOR ( 'NONE', #11981, 1000.000000000000000 ) ;
#19007=VERTEX_POINT ( 'NONE', #22896 ) ;
#19008=ADVANCED_FACE ( 'NONE', ( #12999 ), #7199, .F. ) ;
#19024=ORIENTED_EDGE ( 'NONE', *, *, #11152, .F. ) ;
#19025=CIRCLE ( 'NONE', #901, 0.7500000000000006661 ) ;
#19030=ORIENTED_EDGE ( 'NONE', *, *, #2246, .F. ) ;
#19031=AXIS2_PLACEMENT_3D ( 'NONE', #14148, #10665, #18145 ) ;
#19058=CIRCLE ( 'NONE', #10418, 0.7500000000000006661 ) ;
#19066=ORIENTED_EDGE ( 'NONE', *, *, #4827, .F. ) ;
#19068=LINE ( 'NONE', #9411, #4509 ) ;
#19073=AXIS2_PLACEMENT_3D ( 'NONE', #22292, #4655, #12533 ) ;
#19096=CARTESIAN_POINT ( 'NONE',  ( 44.06606138205700063, 42.82479937715250173, 82.59790614618329130 ) ) ;
#19136=ORIENTED_EDGE ( 'NONE', *, *, #4724, .F. ) ;
#19151=DIRECTION ( 'NONE',  ( 1.000000000000000000, 1.734723475976799945E-16, -1.734723475976814737E-16 ) ) ;
#19155=DIRECTION ( 'NONE',  ( 6.489379976170840313E-31, -1.000000000000000000, 3.491481338843135327E-15 ) ) ;
#19156=CARTESIAN_POINT ( 'NONE',  ( 32.56606138205700773, 40.39281886181299797, 84.30501292736984453 ) ) ;
#19163=CARTESIAN_POINT ( 'NONE',  ( 31.81606138205700418, -39.60718113818700203, 82.55501292737012875 ) ) ;
#19166=CARTESIAN_POINT ( 'NONE',  ( 32.56606138205700773, 40.39281886181299797, 82.55501292736983032 ) ) ;
#19168=DIRECTION ( 'NONE',  ( -1.000000000000000000, -2.065146995210479765E-16, 1.734723475976814737E-16 ) ) ;
#19175=ADVANCED_FACE ( 'NONE', ( #23398 ), #7447, .F. ) ;
#19176=ORIENTED_EDGE ( 'NONE', *, *, #5117, .T. ) ;
#19182=( LENGTH_UNIT ( ) NAMED_UNIT ( * ) SI_UNIT ( .MILLI., .METRE. ) );
#19194=DIRECTION ( 'NONE',  ( 0.000000000000000000, 1.000000000000000000, -4.625929269271481378E-15 ) ) ;
#19200=VERTEX_POINT ( 'NONE', #17363 ) ;
#19218=FACE_OUTER_BOUND ( 'NONE', #5878, .T. ) ;
#19219=CARTESIAN_POINT ( 'NONE',  ( 35.14099152588522657, 1.392818861812999964, 84.30501292737000085 ) ) ;
#19229=CARTESIAN_POINT ( 'NONE',  ( 44.81606138205700063, 40.39281886181299797, 82.55501292736983032 ) ) ;
#19231=EDGE_LOOP ( 'NONE', ( #8553, #16285, #11935, #24339 ) ) ;
#19245=VECTOR ( 'NONE', #7791, 1000.000000000000000 ) ;
#19254=CARTESIAN_POINT ( 'NONE',  ( 44.81606138205700063, -36.05876147765410877, 70.30501292737000085 ) ) ;
#19258=ORIENTED_EDGE ( 'NONE', *, *, #729, .T. ) ;
#19261=CARTESIAN_POINT ( 'NONE',  ( 30.81606138205700418, 0.3928188618129990761, 122.0250129273699997 ) ) ;
#19265=AXIS2_PLACEMENT_3D ( 'NONE', #3792, #11301, #9363 ) ;
#19282=ORIENTED_EDGE ( 'NONE', *, *, #1451, .T. ) ;
#19285=DIRECTION ( 'NONE',  ( 0.000000000000000000, 1.000000000000000000, 0.000000000000000000 ) ) ;
#19293=ADVANCED_FACE ( 'NONE', ( #7835 ), #21350, .F. ) ;
#19295=ORIENTED_EDGE ( 'NONE', *, *, #13016, .F. ) ;
#19301=AXIS2_PLACEMENT_3D ( 'NONE', #22501, #9254, #4985 ) ;
#19309=DIRECTION ( 'NONE',  ( 6.505213034913089466E-17, -1.000000000000000000, 3.491481338843135327E-15 ) ) ;
#19323=EDGE_CURVE ( 'NONE', #23758, #3863, #15681, .T. ) ;
#19326=EDGE_CURVE ( 'NONE', #16812, #21490, #13761, .T. ) ;
#19341=DIRECTION ( 'NONE',  ( 0.000000000000000000, 1.000000000000000000, 0.000000000000000000 ) ) ;
#19345=CYLINDRICAL_SURFACE ( 'NONE', #2334, 1.500000000000001332 ) ;
#19346=VECTOR ( 'NONE', #24157, 1000.000000000000000 ) ;
#19350=CARTESIAN_POINT ( 'NONE',  ( 45.81606138205700063, 39.39281886181299797, 81.75501292736983316 ) ) ;
#19360=ORIENTED_EDGE ( 'NONE', *, *, #16077, .T. ) ;
#19362=VERTEX_POINT ( 'NONE', #14013 ) ;
#19363=CARTESIAN_POINT ( 'NONE',  ( 30.81606138205700418, -38.55876147765410167, 72.21586839016130455 ) ) ;
#19372=EDGE_LOOP ( 'NONE', ( #11341, #9627, #4906, #7842 ) ) ;
#19378=ORIENTED_EDGE ( 'NONE', *, *, #3773, .F. ) ;
#19389=EDGE_LOOP ( 'NONE', ( #3799, #12246, #9655, #3868 ) ) ;
#19391=ORIENTED_EDGE ( 'NONE', *, *, #18197, .T. ) ;
#19400=ORIENTED_EDGE ( 'NONE', *, *, #13016, .T. ) ;
#19401=CARTESIAN_POINT ( 'NONE',  ( 41.14099152588523367, 1.392818861812999964, 93.30501292736998664 ) ) ;
#19410=DIRECTION ( 'NONE',  ( 0.000000000000000000, -1.000000000000000000, 3.304235192336775512E-15 ) ) ;
#19415=CARTESIAN_POINT ( 'NONE',  ( 35.14099152588522657, 40.39281886181299797, 84.30501292736984453 ) ) ;
#19421=ORIENTED_EDGE ( 'NONE', *, *, #11969, .F. ) ;
#19424=SURFACE_STYLE_FILL_AREA ( #3465 ) ;
#19431=CARTESIAN_POINT ( 'NONE',  ( 31.81606138205700418, 40.39281886181299797, 66.30501292737000085 ) ) ;
#19439=CIRCLE ( 'NONE', #8359, 1.750000000000001554 ) ;
#19445=VECTOR ( 'NONE', #18341, 1000.000000000000000 ) ;
#19452=EDGE_CURVE ( 'NONE', #16039, #17020, #15811, .T. ) ;
#19462=AXIS2_PLACEMENT_3D ( 'NONE', #9384, #23392, #1747 ) ;
#19470=CARTESIAN_POINT ( 'NONE',  ( 45.81606138205700063, -34.55876147765410167, 70.30501292737000085 ) ) ;
#19472=DIRECTION ( 'NONE',  ( 0.000000000000000000, 1.000000000000000000, 0.000000000000000000 ) ) ;
#19486=ORIENTED_EDGE ( 'NONE', *, *, #20058, .T. ) ;
#19489=DIRECTION ( 'NONE',  ( 0.000000000000000000, 0.000000000000000000, 1.000000000000000000 ) ) ;
#19492=CARTESIAN_POINT ( 'NONE',  ( 40.64099152588523367, 1.142818861812999742, 93.30501292736998664 ) ) ;
#19494=EDGE_CURVE ( 'NONE', #7168, #13296, #6931, .T. ) ;
#19518=DIRECTION ( 'NONE',  ( 0.000000000000000000, 0.000000000000000000, -1.000000000000000000 ) ) ;
#19532=EDGE_LOOP ( 'NONE', ( #16530, #14367, #959, #13442, #9992, #17203, #21205, #13006, #23250, #24746, #755, #19258, #8313, #1335, #21621, #24 ) ) ;
#19554=CARTESIAN_POINT ( 'NONE',  ( 44.81606138205700063, 34.87886987267150118, 84.30501292736984453 ) ) ;
#19569=CARTESIAN_POINT ( 'NONE',  ( 44.81606138205700063, -3.831401139557048197, 80.75501292737000369 ) ) ;
#19571=EDGE_CURVE ( 'NONE', #11291, #12560, #22619, .T. ) ;
#19573=DIRECTION ( 'NONE',  ( 0.000000000000000000, 1.000000000000000000, -2.775557561562891351E-15 ) ) ;
#19579=ORIENTED_EDGE ( 'NONE', *, *, #10698, .T. ) ;
#19582=EDGE_CURVE ( 'NONE', #25398, #7168, #7033, .T. ) ;
#19599=DIRECTION ( 'NONE',  ( 0.000000000000000000, -1.000000000000000000, 0.000000000000000000 ) ) ;
#19607=VECTOR ( 'NONE', #8816, 1000.000000000000000 ) ;
#19609=ORIENTED_EDGE ( 'NONE', *, *, #9425, .F. ) ;
#19612=LINE ( 'NONE', #21296, #20560 ) ;
#19653=VECTOR ( 'NONE', #12747, 1000.000000000000000 ) ;
#19663=ADVANCED_FACE ( 'NONE', ( #13354 ), #7291, .T. ) ;
#19664=LINE ( 'NONE', #20518, #5131 ) ;
#19670=DIRECTION ( 'NONE',  ( -1.734723475976804876E-16, -3.491481338843135327E-15, -1.000000000000000000 ) ) ;
#19673=AXIS2_PLACEMENT_3D ( 'NONE', #22108, #14136, #10020 ) ;
#19674=DIRECTION ( 'NONE',  ( -1.301042606982603842E-16, 0.000000000000000000, -1.000000000000000000 ) ) ;
#19688=DIRECTION ( 'NONE',  ( 0.000000000000000000, 1.000000000000000000, -2.775557561562891351E-15 ) ) ;
#19690=SURFACE_STYLE_FILL_AREA ( #24271 ) ;
#19696=DIRECTION ( 'NONE',  ( -1.000000000000000000, -2.168404344971010101E-16, 1.734723475976814737E-16 ) ) ;
#19711=ORIENTED_EDGE ( 'NONE', *, *, #14823, .F. ) ;
#19715=ADVANCED_FACE ( 'NONE', ( #11548 ), #13229, .F. ) ;
#19723=AXIS2_PLACEMENT_3D ( 'NONE', #4777, #10332, #16494 ) ;
#19751=FACE_OUTER_BOUND ( 'NONE', #8098, .T. ) ;
#19762=CARTESIAN_POINT ( 'NONE',  ( 38.38987944808049235, -39.60718113818700203, 84.30501292737011454 ) ) ;
#19763=EDGE_CURVE ( 'NONE', #23326, #16761, #330, .T. ) ;
#19771=LINE ( 'NONE', #11930, #23823 ) ;
#19786=DIRECTION ( 'NONE',  ( 0.000000000000000000, 1.000000000000000000, -3.469446951953614189E-15 ) ) ;
#19788=ORIENTED_EDGE ( 'NONE', *, *, #20592, .T. ) ;
#19803=CARTESIAN_POINT ( 'NONE',  ( 34.56606138205700773, 45.04446929126255128, 81.37823623207320622 ) ) ;
#19809=VERTEX_POINT ( 'NONE', #23368 ) ;
#19811=ORIENTED_EDGE ( 'NONE', *, *, #6322, .T. ) ;
#19838=CARTESIAN_POINT ( 'NONE',  ( 44.81606138205700063, 40.34464305740947765, 81.44836866983821722 ) ) ;
#19845=VECTOR ( 'NONE', #1908, 1000.000000000000000 ) ;
#19847=DIRECTION ( 'NONE',  ( -1.734723475976809806E-16, 0.000000000000000000, -1.000000000000000000 ) ) ;
#19853=CARTESIAN_POINT ( 'NONE',  ( 45.81606138205700063, -34.55876147765410167, 70.30501292737000085 ) ) ;
#19860=LINE ( 'NONE', #2202, #23033 ) ;
#19869=ADVANCED_FACE ( 'NONE', ( #8056 ), #21956, .T. ) ;
#19908=AXIS2_PLACEMENT_3D ( 'NONE', #5154, #16876, #18936 ) ;
#19913=CARTESIAN_POINT ( 'NONE',  ( 44.81606138205700063, -26.74044063519535186, 82.50501292737007475 ) ) ;
#19926=ORIENTED_EDGE ( 'NONE', *, *, #23565, .T. ) ;
#19947=CARTESIAN_POINT ( 'NONE',  ( 44.81606138205700063, 40.39281886181299797, 80.75501292736983316 ) ) ;
#19950=ORIENTED_EDGE ( 'NONE', *, *, #4557, .T. ) ;
#19951=DIRECTION ( 'NONE',  ( 1.734723475976814737E-16, -1.000000000000000000, 3.491481338843135327E-15 ) ) ;
#19957=CYLINDRICAL_SURFACE ( 'NONE', #5856, 1.500000000000001332 ) ;
#19961=EDGE_CURVE ( 'NONE', #10371, #24890, #178, .T. ) ;
#19984=DIRECTION ( 'NONE',  ( -1.734723475976809806E-16, 1.000000000000000000, -3.269436733918100469E-15 ) ) ;
#20005=DIRECTION ( 'NONE',  ( -1.000000000000000000, 6.018531076210110289E-31, 1.734723475976804876E-16 ) ) ;
#20042=CIRCLE ( 'NONE', #23718, 12.59999999999999964 ) ;
#20050=ORIENTED_EDGE ( 'NONE', *, *, #22810, .T. ) ;
#20058=EDGE_CURVE ( 'NONE', #194, #131, #22168, .T. ) ;
#20077=AXIS2_PLACEMENT_3D ( 'NONE', #14633, #16820, #7030 ) ;
#20080=CARTESIAN_POINT ( 'NONE',  ( 35.64099152588522657, 0.3928188618129990761, 80.05501292736997243 ) ) ;
#20096=EDGE_CURVE ( 'NONE', #3821, #1971, #2861, .T. ) ;
#20101=FACE_OUTER_BOUND ( 'NONE', #7146, .T. ) ;
#20110=CARTESIAN_POINT ( 'NONE',  ( 32.56606138205700773, 43.35512946304240245, 81.37823623207322044 ) ) ;
#20126=ORIENTED_EDGE ( 'NONE', *, *, #666, .F. ) ;
#20127=CARTESIAN_POINT ( 'NONE',  ( 45.81606138205700063, -11.72563467517899838, 72.98595903681223263 ) ) ;
#20142=LINE ( 'NONE', #2230, #18842 ) ;
#20171=DIRECTION ( 'NONE',  ( 0.000000000000000000, -1.000000000000000000, 0.000000000000000000 ) ) ;
#20174=CARTESIAN_POINT ( 'NONE',  ( 30.81606138205700418, 0.1601050959395486362, 68.80395113470939350 ) ) ;
#20175=VERTEX_POINT ( 'NONE', #6870 ) ;
#20212=AXIS2_PLACEMENT_3D ( 'NONE', #8455, #4460, #20171 ) ;
#20213=CARTESIAN_POINT ( 'NONE',  ( 31.81606138205700418, -33.05876147765410167, 70.30501292737000085 ) ) ;
#20226=LINE ( 'NONE', #2565, #12157 ) ;
#20238=CARTESIAN_POINT ( 'NONE',  ( 38.41621794735363693, -36.60729675983900222, 84.30501292737011454 ) ) ;
#20247=FACE_OUTER_BOUND ( 'NONE', #7139, .T. ) ;
#20257=ORIENTED_EDGE ( 'NONE', *, *, #17120, .T. ) ;
#20258=AXIS2_PLACEMENT_3D ( 'NONE', #15700, #21128, #21632 ) ;
#20265=DIRECTION ( 'NONE',  ( 1.000000000000000000, 2.168404344971055214E-16, -1.734723475976814737E-16 ) ) ;
#20267=AXIS2_PLACEMENT_3D ( 'NONE', #11675, #21075, #21447 ) ;
#20290=ORIENTED_EDGE ( 'NONE', *, *, #6950, .F. ) ;
#20306=( NAMED_UNIT ( * ) SI_UNIT ( $, .STERADIAN. ) SOLID_ANGLE_UNIT ( ) );
#20316=VECTOR ( 'NONE', #11512, 1000.000000000000000 ) ;
#20354=FACE_OUTER_BOUND ( 'NONE', #9617, .T. ) ;
#20361=EDGE_CURVE ( 'NONE', #22752, #20175, #3511, .T. ) ;
#20366=LINE ( 'NONE', #10456, #3082 ) ;
#20382=DIRECTION ( 'NONE',  ( -1.000000000000000000, -1.734723475976804876E-16, 1.734723475976814737E-16 ) ) ;
#20396=CARTESIAN_POINT ( 'NONE',  ( 32.56606138205700773, 43.04446929126255128, 81.37823623207322044 ) ) ;
#20405=ORIENTED_EDGE ( 'NONE', *, *, #1219, .F. ) ;
#20414=ORIENTED_EDGE ( 'NONE', *, *, #2321, .T. ) ;
#20421=SURFACE_STYLE_USAGE ( .BOTH. , #11850 ) ;
#20429=DIRECTION ( 'NONE',  ( -2.453269466693404537E-16, 0.7071067811865489050, -0.7071067811865460184 ) ) ;
#20433=FACE_BOUND ( 'NONE', #21295, .T. ) ;
#20439=CARTESIAN_POINT ( 'NONE',  ( 45.81606138205700063, 31.19260082947834078, 104.9690409559304101 ) ) ;
#20441=EDGE_LOOP ( 'NONE', ( #22339, #3954, #15786, #21652 ) ) ;
#20450=ORIENTED_EDGE ( 'NONE', *, *, #12738, .F. ) ;
#20459=CARTESIAN_POINT ( 'NONE',  ( 44.81606138205700063, 31.19260082947834078, 104.9690409559304101 ) ) ;
#20460=VECTOR ( 'NONE', #17283, 1000.000000000000000 ) ;
#20477=LINE ( 'NONE', #2939, #18840 ) ;
#20507=DIRECTION ( 'NONE',  ( 0.000000000000000000, -3.965082230804126670E-15, -1.000000000000000000 ) ) ;
#20513=CARTESIAN_POINT ( 'NONE',  ( 32.56606138205700773, 47.04446929126254417, 81.37823623207319201 ) ) ;
#20518=CARTESIAN_POINT ( 'NONE',  ( 15.14989484155900001, 36.04731275961434989, 83.30501292736985874 ) ) ;
#20520=LINE ( 'NONE', #18586, #19607 ) ;
#20522=CARTESIAN_POINT ( 'NONE',  ( 44.06606138205700063, 43.35512946304240245, 83.12823623207320622 ) ) ;
#20526=AXIS2_PLACEMENT_3D ( 'NONE', #6677, #14792, #24308 ) ;
#20535=ORIENTED_EDGE ( 'NONE', *, *, #11009, .T. ) ;
#20540=VECTOR ( 'NONE', #3472, 1000.000000000000000 ) ;
#20543=ORIENTED_EDGE ( 'NONE', *, *, #13692, .T. ) ;
#20553=EDGE_LOOP ( 'NONE', ( #4073, #7567, #10101, #14669 ) ) ;
#20560=VECTOR ( 'NONE', #11524, 1000.000000000000000 ) ;
#20561=AXIS2_PLACEMENT_3D ( 'NONE', #7523, #5459, #19489 ) ;
#20570=ORIENTED_EDGE ( 'NONE', *, *, #15871, .F. ) ;
#20583=VECTOR ( 'NONE', #11584, 1000.000000000000000 ) ;
#20588=CARTESIAN_POINT ( 'NONE',  ( 32.56606138205700773, 40.92314894770289158, 83.08534301325974525 ) ) ;
#20592=EDGE_CURVE ( 'NONE', #5274, #22820, #9443, .T. ) ;
#20599=EDGE_CURVE ( 'NONE', #5938, #21676, #12783, .T. ) ;
#20601=UNCERTAINTY_MEASURE_WITH_UNIT (LENGTH_MEASURE( 1.000000000000000082E-05 ), #21242, 'distance_accuracy_value', 'NONE');
#20602=AXIS2_PLACEMENT_3D ( 'NONE', #10405, #4482, #23790 ) ;
#20613=ADVANCED_FACE ( 'NONE', ( #22047 ), #4408, .F. ) ;
#20632=ORIENTED_EDGE ( 'NONE', *, *, #2521, .T. ) ;
#20656=AXIS2_PLACEMENT_3D ( 'NONE', #22437, #5401, #25206 ) ;
#20669=DIRECTION ( 'NONE',  ( -1.734723475976804876E-16, -3.469446951953610245E-15, -1.000000000000000000 ) ) ;
#20675=LINE ( 'NONE', #1338, #22749 ) ;
#20708=AXIS2_PLACEMENT_3D ( 'NONE', #24277, #12467, #7026 ) ;
#20738=PLANE ( 'NONE',  #9922 ) ;
#20740=EDGE_LOOP ( 'NONE', ( #14872, #12325, #4593, #12987 ) ) ;
#20757=PLANE ( 'NONE',  #14157 ) ;
#20770=VERTEX_POINT ( 'NONE', #17146 ) ;
#20777=DIRECTION ( 'NONE',  ( -1.734723475976814737E-16, 0.000000000000000000, -1.000000000000000000 ) ) ;
#20783=DIRECTION ( 'NONE',  ( 0.000000000000000000, -3.491481338843135327E-15, -1.000000000000000000 ) ) ;
#20786=PLANE ( 'NONE',  #17846 ) ;
#20791=LINE ( 'NONE', #3126, #5488 ) ;
#20799=ORIENTED_EDGE ( 'NONE', *, *, #9100, .T. ) ;
#20818=ORIENTED_EDGE ( 'NONE', *, *, #9414, .F. ) ;
#20829=CARTESIAN_POINT ( 'NONE',  ( 30.81606138205700418, -34.55876147765410167, 70.30501292737000085 ) ) ;
#20840=LINE ( 'NONE', #14650, #8759 ) ;
#20846=LINE ( 'NONE', #1257, #3186 ) ;
#20850=CYLINDRICAL_SURFACE ( 'NONE', #20526, 3.000000000000002665 ) ;
#20851=ORIENTED_EDGE ( 'NONE', *, *, #19326, .T. ) ;
#20899=LINE ( 'NONE', #11113, #9225 ) ;
#20907=VECTOR ( 'NONE', #12477, 1000.000000000000000 ) ;
#20910=FACE_OUTER_BOUND ( 'NONE', #11731, .T. ) ;
#20914=CARTESIAN_POINT ( 'NONE',  ( 45.81606138205700063, -25.52563857111379875, 92.39878177866870601 ) ) ;
#20923=DIRECTION ( 'NONE',  ( 1.734723475976814737E-16, -1.000000000000000000, 3.491481338843135327E-15 ) ) ;
#20924=DIRECTION ( 'NONE',  ( 1.734723475976814737E-16, -1.000000000000000000, 3.491481338843135327E-15 ) ) ;
#20938=VERTEX_POINT ( 'NONE', #23300 ) ;
#20944=CARTESIAN_POINT ( 'NONE',  ( 31.81606138205700418, -26.74044063519535186, 82.55501292737007191 ) ) ;
#20947=ORIENTED_EDGE ( 'NONE', *, *, #3958, .F. ) ;
#20951=CARTESIAN_POINT ( 'NONE',  ( 30.81606138205700418, 40.39281886181299797, 83.30501292736984453 ) ) ;
#20957=ORIENTED_EDGE ( 'NONE', *, *, #1674, .F. ) ;
#20999=ORIENTED_EDGE ( 'NONE', *, *, #1598, .F. ) ;
#21005=CARTESIAN_POINT ( 'NONE',  ( 38.41621794735363693, -36.60729675983900222, 84.30501292737011454 ) ) ;
#21018=EDGE_LOOP ( 'NONE', ( #7236, #4171, #11151, #5302 ) ) ;
#21027=FACE_OUTER_BOUND ( 'NONE', #89, .T. ) ;
#21028=DIRECTION ( 'NONE',  ( 1.000000000000000000, 1.734723475976804876E-16, -1.734723475976814737E-16 ) ) ;
#21036=VERTEX_POINT ( 'NONE', #18167 ) ;
#21038=DIRECTION ( 'NONE',  ( 1.734723475976814737E-16, -1.000000000000000000, 3.491481338843135327E-15 ) ) ;
#21053=DIRECTION ( 'NONE',  ( 2.156013462999745228E-15, -1.000000000000000000, 3.491481338843135327E-15 ) ) ;
#21066=ORIENTED_EDGE ( 'NONE', *, *, #23336, .T. ) ;
#21069=DIRECTION ( 'NONE',  ( 0.000000000000000000, -1.000000000000000000, 3.469446951953617344E-15 ) ) ;
#21072=VECTOR ( 'NONE', #975, 1000.000000000000000 ) ;
#21075=DIRECTION ( 'NONE',  ( 1.734723475976804876E-16, 3.496552006265755350E-15, 1.000000000000000000 ) ) ;
#21103=AXIS2_PLACEMENT_3D ( 'NONE', #15645, #9736, #23243 ) ;
#21107=AXIS2_PLACEMENT_3D ( 'NONE', #3914, #9721, #7657 ) ;
#21122=CARTESIAN_POINT ( 'NONE',  ( 45.81606138205700063, -3.831401139557048197, 80.75501292737000369 ) ) ;
#21124=CIRCLE ( 'NONE', #2603, 3.999999999999996447 ) ;
#21128=DIRECTION ( 'NONE',  ( 2.595751990468335074E-30, 1.000000000000000000, -3.491481338843135327E-15 ) ) ;
#21130=COLOUR_RGB ( '', 0.40784314, 0.44705882, 0.49803922) ;
#21141=EDGE_LOOP ( 'NONE', ( #11011, #16898, #10352, #6002 ) ) ;
#21153=DIRECTION ( 'NONE',  ( -0.9681609007195522976, 0.2503287245161955887, -7.060689259245944321E-16 ) ) ;
#21180=AXIS2_PLACEMENT_3D ( 'NONE', #15221, #22700, #20783 ) ;
#21192=CIRCLE ( 'NONE', #8030, 0.7500000000000006661 ) ;
#21199=EDGE_LOOP ( 'NONE', ( #21336, #12357, #10790, #6887 ) ) ;
#21205=ORIENTED_EDGE ( 'NONE', *, *, #243, .T. ) ;
#21212=ORIENTED_EDGE ( 'NONE', *, *, #19961, .T. ) ;
#21226=DIRECTION ( 'NONE',  ( -1.000000000000000000, 6.018531076210120799E-31, 1.734723475976804876E-16 ) ) ;
#21231=CARTESIAN_POINT ( 'NONE',  ( 44.06606138205700063, 40.39281886181299797, 82.55501292736983032 ) ) ;
#21234=CARTESIAN_POINT ( 'NONE',  ( 31.81606138205700418, -26.74044063519544778, 66.30501292737000085 ) ) ;
#21240=EDGE_CURVE ( 'NONE', #16610, #22911, #10939, .T. ) ;
#21242=( LENGTH_UNIT ( ) NAMED_UNIT ( * ) SI_UNIT ( .MILLI., .METRE. ) );
#21255=ORIENTED_EDGE ( 'NONE', *, *, #3584, .T. ) ;
#21264=EDGE_LOOP ( 'NONE', ( #5838, #8070, #2240, #15889 ) ) ;
#21268=VECTOR ( 'NONE', #548, 1000.000000000000114 ) ;
#21276=CARTESIAN_POINT ( 'NONE',  ( 31.81606138205700418, 40.39281886181299797, 82.55501292736983032 ) ) ;
#21279=PLANE ( 'NONE',  #13460 ) ;
#21281=DIRECTION ( 'NONE',  ( 2.453269466693404537E-16, -0.7071067811865489050, 0.7071067811865460184 ) ) ;
#21295=EDGE_LOOP ( 'NONE', ( #25401, #10979, #9227, #3903, #4380, #3288, #10629, #9527 ) ) ;
#21296=CARTESIAN_POINT ( 'NONE',  ( 35.64099152588522657, 40.39281886181299797, 84.30501292736984453 ) ) ;
#21312=ORIENTED_EDGE ( 'NONE', *, *, #8068, .T. ) ;
#21314=FACE_OUTER_BOUND ( 'NONE', #24628, .T. ) ;
#21315=DIRECTION ( 'NONE',  ( -1.000000000000000000, -1.734723475976804876E-16, 1.734723475976814737E-16 ) ) ;
#21323=EDGE_LOOP ( 'NONE', ( #272, #8754, #24986, #9928 ) ) ;
#21325=DIRECTION ( 'NONE',  ( 1.000000000000000000, 1.734723475976804876E-16, -1.734723475976814737E-16 ) ) ;
#21336=ORIENTED_EDGE ( 'NONE', *, *, #12903, .T. ) ;
#21340=DIRECTION ( 'NONE',  ( 1.734723475976804876E-16, 3.491481338843135327E-15, 1.000000000000000000 ) ) ;
#21348=EDGE_CURVE ( 'NONE', #7324, #7168, #55, .T. ) ;
#21350=CYLINDRICAL_SURFACE ( 'NONE', #9403, 0.7500000000000006661 ) ;
#21369=VECTOR ( 'NONE', #10909, 1000.000000000000000 ) ;
#21374=ADVANCED_FACE ( 'NONE', ( #23639 ), #15783, .T. ) ;
#21379=DIRECTION ( 'NONE',  ( 1.734723475976814737E-16, -1.000000000000000000, 3.491481338843135327E-15 ) ) ;
#21390=VERTEX_POINT ( 'NONE', #11934 ) ;
#21409=DIRECTION ( 'NONE',  ( -8.381647117973248681E-31, -0.7071067811865460184, -0.7071067811865489050 ) ) ;
#21415=CARTESIAN_POINT ( 'NONE',  ( 44.06606138205700063, 40.92314894770294842, 83.08534301325974525 ) ) ;
#21419=DIRECTION ( 'NONE',  ( 1.734723475976814737E-16, -1.000000000000000000, 3.491481338843135327E-15 ) ) ;
#21429=VERTEX_POINT ( 'NONE', #21834 ) ;
#21433=VERTEX_POINT ( 'NONE', #10367 ) ;
#21447=DIRECTION ( 'NONE',  ( 0.000000000000000000, 1.000000000000000000, -6.938893903907222067E-15 ) ) ;
#21462=EDGE_LOOP ( 'NONE', ( #24146, #13927, #10129, #19360 ) ) ;
#21470=EDGE_CURVE ( 'NONE', #7305, #13947, #14481, .T. ) ;
#21484=AXIS2_PLACEMENT_3D ( 'NONE', #19947, #2282, #23286 ) ;
#21485=DIRECTION ( 'NONE',  ( -6.505213034913079606E-17, 1.000000000000000000, -3.491481338843135327E-15 ) ) ;
#21490=VERTEX_POINT ( 'NONE', #10625 ) ;
#21496=ORIENTED_EDGE ( 'NONE', *, *, #458, .T. ) ;
#21506=CARTESIAN_POINT ( 'NONE',  ( 30.81606138205700773, 40.39281886181299797, 81.44836866983821722 ) ) ;
#21519=VECTOR ( 'NONE', #12841, 1000.000000000000000 ) ;
#21536=EDGE_CURVE ( 'NONE', #14213, #17064, #23338, .T. ) ;
#21543=CIRCLE ( 'NONE', #24811, 1.750000000000001554 ) ;
#21551=CIRCLE ( 'NONE', #25219, 1.500000000000001332 ) ;
#21559=AXIS2_PLACEMENT_3D ( 'NONE', #20238, #9042, #12779 ) ;
#21581=ORIENTED_EDGE ( 'NONE', *, *, #18535, .T. ) ;
#21590=ORIENTED_EDGE ( 'NONE', *, *, #16006, .T. ) ;
#21592=ORIENTED_EDGE ( 'NONE', *, *, #10045, .F. ) ;
#21613=FACE_OUTER_BOUND ( 'NONE', #25141, .T. ) ;
#21621=ORIENTED_EDGE ( 'NONE', *, *, #13097, .T. ) ;
#21632=DIRECTION ( 'NONE',  ( -1.000000000000000000, 0.000000000000000000, 0.000000000000000000 ) ) ;
#21652=ORIENTED_EDGE ( 'NONE', *, *, #721, .T. ) ;
#21676=VERTEX_POINT ( 'NONE', #395 ) ;
#21678=VERTEX_POINT ( 'NONE', #19 ) ;
#21679=PLANE ( 'NONE',  #20561 ) ;
#21686=EDGE_CURVE ( 'NONE', #4432, #7783, #152, .T. ) ;
#21688=DIRECTION ( 'NONE',  ( 1.000000000000000000, 1.734723475976805122E-16, -1.734723475976811039E-16 ) ) ;
#21711=VERTEX_POINT ( 'NONE', #21802 ) ;
#21712=VECTOR ( 'NONE', #2842, 1000.000000000000114 ) ;
#21715=VECTOR ( 'NONE', #6483, 1000.000000000000000 ) ;
#21735=FACE_OUTER_BOUND ( 'NONE', #11067, .T. ) ;
#21737=CYLINDRICAL_SURFACE ( 'NONE', #24632, 1.000000000000000888 ) ;
#21738=CARTESIAN_POINT ( 'NONE',  ( 45.81606138205700063, 40.39281886181299797, 82.55501292736983032 ) ) ;
#21740=DIRECTION ( 'NONE',  ( 1.000000000000000000, 1.734723475976804876E-16, -1.734723475976814737E-16 ) ) ;
#21750=VECTOR ( 'NONE', #5899, 1000.000000000000000 ) ;
#21771=LINE ( 'NONE', #19838, #5765 ) ;
#21778=ORIENTED_EDGE ( 'NONE', *, *, #12729, .F. ) ;
#21784=DIRECTION ( 'NONE',  ( 1.000000000000000000, 1.734723475976804876E-16, -1.734723475976814737E-16 ) ) ;
#21793=VECTOR ( 'NONE', #20923, 1000.000000000000000 ) ;
#21802=CARTESIAN_POINT ( 'NONE',  ( 44.06606138205700063, 45.04446929126260102, 81.37823623207320622 ) ) ;
#21804=ORIENTED_EDGE ( 'NONE', *, *, #4724, .T. ) ;
#21811=ORIENTED_EDGE ( 'NONE', *, *, #261, .F. ) ;
#21813=DIRECTION ( 'NONE',  ( 0.000000000000000000, -1.000000000000000000, 3.469446951953701358E-15 ) ) ;
#21820=EDGE_LOOP ( 'NONE', ( #17189, #3947, #16258, #3588 ) ) ;
#21821=LINE ( 'NONE', #12049, #10850 ) ;
#21832=EDGE_LOOP ( 'NONE', ( #18414, #14147 ) ) ;
#21834=CARTESIAN_POINT ( 'NONE',  ( 32.56606138205700773, 45.04446929126260102, 82.37823623207320622 ) ) ;
#21835=ORIENTED_EDGE ( 'NONE', *, *, #13175, .F. ) ;
#21843=ORIENTED_EDGE ( 'NONE', *, *, #8465, .T. ) ;
#21846=CARTESIAN_POINT ( 'NONE',  ( 44.06606138205700063, 45.04446929126260102, 81.37823623207320622 ) ) ;
#21848=ADVANCED_FACE ( 'NONE', ( #20247 ), #14325, .T. ) ;
#21856=AXIS2_PLACEMENT_3D ( 'NONE', #11172, #3163, #6915 ) ;
#21858=EDGE_CURVE ( 'NONE', #16039, #1577, #6592, .T. ) ;
#21864=CARTESIAN_POINT ( 'NONE',  ( 30.81606138205700418, 40.83281886181300280, 78.30501292736983032 ) ) ;
#21866=ADVANCED_FACE ( 'NONE', ( #903, #6715 ), #648, .F. ) ;
#21871=VERTEX_POINT ( 'NONE', #16368 ) ;
#21873=ORIENTED_EDGE ( 'NONE', *, *, #15538, .T. ) ;
#21890=LINE ( 'NONE', #18036, #25455 ) ;
#21897=LINE ( 'NONE', #6558, #17720 ) ;
#21915=AXIS2_PLACEMENT_3D ( 'NONE', #3582, #25211, #19688 ) ;
#21929=AXIS2_PLACEMENT_3D ( 'NONE', #10651, #18500, #6899 ) ;
#21934=FACE_OUTER_BOUND ( 'NONE', #5654, .T. ) ;
#21935=CARTESIAN_POINT ( 'NONE',  ( 30.81606138205700418, 40.39281886181299797, 82.55501292736983032 ) ) ;
#21949=CARTESIAN_POINT ( 'NONE',  ( 44.81606138205700063, -11.72563467517899838, 72.98595903681223263 ) ) ;
#21956=PLANE ( 'NONE',  #14760 ) ;
#21965=ORIENTED_EDGE ( 'NONE', *, *, #128, .T. ) ;
#21966=CARTESIAN_POINT ( 'NONE',  ( 45.81606138205700063, -38.55876147765410167, 72.21586839016147508 ) ) ;
#21970=ORIENTED_EDGE ( 'NONE', *, *, #23908, .F. ) ;
#21972=DIRECTION ( 'NONE',  ( 0.000000000000000000, 1.000000000000000000, -3.469446951953614189E-15 ) ) ;
#21973=DIRECTION ( 'NONE',  ( 0.000000000000000000, 0.7071067811865455743, 0.7071067811865494601 ) ) ;
#21982=VECTOR ( 'NONE', #7147, 1000.000000000000000 ) ;
#21999=EDGE_CURVE ( 'NONE', #7140, #24390, #3096, .T. ) ;
#22013=DIRECTION ( 'NONE',  ( -1.000000000000000000, -1.734723475976804876E-16, 1.734723475976814737E-16 ) ) ;
#22014=DIRECTION ( 'NONE',  ( 0.000000000000000000, 1.000000000000000000, 0.000000000000000000 ) ) ;
#22016=DIRECTION ( 'NONE',  ( 1.000000000000000000, 1.734723475976804876E-16, -1.734723475976814737E-16 ) ) ;
#22029=CIRCLE ( 'NONE', #23254, 2.000000000000001776 ) ;
#22032=FACE_OUTER_BOUND ( 'NONE', #23450, .T. ) ;
#22036=CARTESIAN_POINT ( 'NONE',  ( 38.41621794735363693, -36.60729675983900222, 84.30501292737011454 ) ) ;
#22047=FACE_OUTER_BOUND ( 'NONE', #22657, .T. ) ;
#22059=DIRECTION ( 'NONE',  ( -1.734723475976804876E-16, -3.491481338843135327E-15, -1.000000000000000000 ) ) ;
#22074=DIRECTION ( 'NONE',  ( -1.734723475976879818E-16, 1.000000000000000000, -4.343580702399009298E-14 ) ) ;
#22077=DIRECTION ( 'NONE',  ( 1.510383499235849534E-16, 0.1218693434051499741, 0.9925461516413217611 ) ) ;
#22083=VERTEX_POINT ( 'NONE', #10300 ) ;
#22094=VERTEX_POINT ( 'NONE', #20213 ) ;
#22105=ORIENTED_EDGE ( 'NONE', *, *, #6273, .T. ) ;
#22108=CARTESIAN_POINT ( 'NONE',  ( 44.81606138205700063, -34.55876147765410167, 70.30501292737000085 ) ) ;
#22110=CARTESIAN_POINT ( 'NONE',  ( 44.81606138205700063, 0.1601050959395486362, 68.80395113470939350 ) ) ;
#22123=ORIENTED_EDGE ( 'NONE', *, *, #13097, .F. ) ;
#22124=CARTESIAN_POINT ( 'NONE',  ( 44.81606138205700063, -34.55876147765410167, 70.30501292737000085 ) ) ;
#22143=CARTESIAN_POINT ( 'NONE',  ( 45.81606138205700063, 40.34464305740947765, 81.44836866983821722 ) ) ;
#22149=CARTESIAN_POINT ( 'NONE',  ( 35.64099152588522657, -1.357181138186998925, 79.30501292737000085 ) ) ;
#22168=CIRCLE ( 'NONE', #5713, 1.750000000000001554 ) ;
#22180=ORIENTED_EDGE ( 'NONE', *, *, #17059, .T. ) ;
#22190=CARTESIAN_POINT ( 'NONE',  ( 35.64099152588522657, -8.607181138186998481, 78.30501292736998664 ) ) ;
#22195=LINE ( 'NONE', #17839, #7318 ) ;
#22213=ORIENTED_EDGE ( 'NONE', *, *, #19323, .F. ) ;
#22230=EDGE_LOOP ( 'NONE', ( #7268, #9889 ) ) ;
#22232=ORIENTED_EDGE ( 'NONE', *, *, #12234, .T. ) ;
#22238=AXIS2_PLACEMENT_3D ( 'NONE', #337, #4101, #8219 ) ;
#22246=DIRECTION ( 'NONE',  ( -1.000000000000000000, -2.065146995210479765E-16, 1.734723475976814737E-16 ) ) ;
#22247=ADVANCED_FACE ( 'NONE', ( #14658 ), #20850, .T. ) ;
#22263=FACE_OUTER_BOUND ( 'NONE', #3076, .T. ) ;
#22271=CARTESIAN_POINT ( 'NONE',  ( 40.64099152588523367, -8.607181138186998481, 79.30501292737000085 ) ) ;
#22280=DIRECTION ( 'NONE',  ( -1.000000000000000000, -1.734723475976804876E-16, 1.734723475976814737E-16 ) ) ;
#22291=CARTESIAN_POINT ( 'NONE',  ( 45.81606138205700063, -33.05876147765410167, 70.30501292737000085 ) ) ;
#22292=CARTESIAN_POINT ( 'NONE',  ( 30.81606138205700418, 39.39281886181299797, 81.75501292736984738 ) ) ;
#22301=DIRECTION ( 'NONE',  ( -1.734723475976814737E-16, 1.000000000000000000, -3.491481338843135327E-15 ) ) ;
#22304=CIRCLE ( 'NONE', #11201, 1.500000000000001332 ) ;
#22306=VERTEX_POINT ( 'NONE', #24440 ) ;
#22310=EDGE_CURVE ( 'NONE', #21429, #4268, #5002, .T. ) ;
#22314=EDGE_CURVE ( 'NONE', #17064, #13535, #2926, .T. ) ;
#22328=DIRECTION ( 'NONE',  ( -1.734723475976814737E-16, 1.000000000000000000, -3.491481338843135327E-15 ) ) ;
#22339=ORIENTED_EDGE ( 'NONE', *, *, #9290, .F. ) ;
#22362=FACE_OUTER_BOUND ( 'NONE', #12197, .T. ) ;
#22409=DIRECTION ( 'NONE',  ( 0.000000000000000000, 1.000000000000000000, 0.000000000000000000 ) ) ;
#22425=VERTEX_POINT ( 'NONE', #13386 ) ;
#22437=CARTESIAN_POINT ( 'NONE',  ( 17.31606138205699708, 34.87886987267149408, 78.19668729537065133 ) ) ;
#22449=EDGE_CURVE ( 'NONE', #6502, #2759, #17119, .T. ) ;
#22469=DIRECTION ( 'NONE',  ( 0.000000000000000000, 0.000000000000000000, 1.000000000000000000 ) ) ;
#22472=ORIENTED_EDGE ( 'NONE', *, *, #20599, .T. ) ;
#22474=CARTESIAN_POINT ( 'NONE',  ( 44.06606138205700063, 43.35512946304240245, 81.37823623207322044 ) ) ;
#22476=ORIENTED_EDGE ( 'NONE', *, *, #19763, .T. ) ;
#22486=EDGE_CURVE ( 'NONE', #24557, #7305, #13543, .T. ) ;
#22491=EDGE_CURVE ( 'NONE', #10628, #8863, #8214, .T. ) ;
#22501=CARTESIAN_POINT ( 'NONE',  ( 35.64099152588522657, 1.142818861812999742, 82.55501292736997243 ) ) ;
#22536=LINE ( 'NONE', #4887, #24170 ) ;
#22537=DIRECTION ( 'NONE',  ( 1.000000000000000000, 0.000000000000000000, 0.000000000000000000 ) ) ;
#22545=CYLINDRICAL_SURFACE ( 'NONE', #19031, 1.500000000000001332 ) ;
#22561=ORIENTED_EDGE ( 'NONE', *, *, #7515, .T. ) ;
#22572=VECTOR ( 'NONE', #18593, 1000.000000000000000 ) ;
#22578=CARTESIAN_POINT ( 'NONE',  ( 35.64099152588523367, 1.392818861812999964, 93.30501292736998664 ) ) ;
#22595=CARTESIAN_POINT ( 'NONE',  ( 45.81606138205700063, 40.39281886181299797, 84.30501292736984453 ) ) ;
#22604=ORIENTED_EDGE ( 'NONE', *, *, #25171, .F. ) ;
#22609=CARTESIAN_POINT ( 'NONE',  ( 40.64099152588523367, -8.607181138186998481, 88.30501292736998664 ) ) ;
#22615=CARTESIAN_POINT ( 'NONE',  ( 40.64099152588522657, 1.142818861812999742, 84.30501292737000085 ) ) ;
#22619=LINE ( 'NONE', #4975, #2793 ) ;
#22638=EDGE_CURVE ( 'NONE', #19362, #2254, #4602, .T. ) ;
#22640=CARTESIAN_POINT ( 'NONE',  ( 40.64099152588522657, 1.142818861812999742, 82.55501292736997243 ) ) ;
#22657=EDGE_LOOP ( 'NONE', ( #20257, #3974, #22213, #14907 ) ) ;
#22676=CARTESIAN_POINT ( 'NONE',  ( 44.81606138205700063, -25.52563857111379875, 92.39878177866870601 ) ) ;
#22688=ORIENTED_EDGE ( 'NONE', *, *, #25106, .T. ) ;
#22700=DIRECTION ( 'NONE',  ( -1.734723475976814737E-16, 1.000000000000000000, -3.491481338843135327E-15 ) ) ;
#22702=ORIENTED_EDGE ( 'NONE', *, *, #9675, .F. ) ;
#22711=EDGE_CURVE ( 'NONE', #16812, #23473, #2143, .T. ) ;
#22720=CARTESIAN_POINT ( 'NONE',  ( 45.81606138205700063, 40.39281886181299797, 66.30501292737000085 ) ) ;
#22726=CARTESIAN_POINT ( 'NONE',  ( 31.81606138205700418, 40.39281886181299797, 81.75501292736983316 ) ) ;
#22728=VERTEX_POINT ( 'NONE', #2522 ) ;
#22735=VERTEX_POINT ( 'NONE', #6411 ) ;
#22745=LINE ( 'NONE', #6908, #10037 ) ;
#22749=VECTOR ( 'NONE', #10891, 1000.000000000000000 ) ;
#22752=VERTEX_POINT ( 'NONE', #10402 ) ;
#22753=DIRECTION ( 'NONE',  ( 1.734723475976804876E-16, 3.491481338843135327E-15, 1.000000000000000000 ) ) ;
#22763=CARTESIAN_POINT ( 'NONE',  ( 44.81606138205700063, 34.87886987267150118, 81.44836866983821722 ) ) ;
#22772=ADVANCED_FACE ( 'NONE', ( #18266 ), #15931, .F. ) ;
#22803=VECTOR ( 'NONE', #13450, 1000.000000000000000 ) ;
#22804=DIRECTION ( 'NONE',  ( 0.000000000000000000, 1.000000000000000000, -6.938893903907222067E-15 ) ) ;
#22810=EDGE_CURVE ( 'NONE', #15469, #10773, #14513, .T. ) ;
#22815=DIRECTION ( 'NONE',  ( -1.734723475976814737E-16, 1.000000000000000000, -3.491481338843135327E-15 ) ) ;
#22820=VERTEX_POINT ( 'NONE', #14636 ) ;
#22839=SHAPE_DEFINITION_REPRESENTATION ( #17538, #14684 ) ;
#22866=CYLINDRICAL_SURFACE ( 'NONE', #6717, 1.500000000000001332 ) ;
#22870=DIRECTION ( 'NONE',  ( 1.000000000000000000, 1.734723475976804876E-16, -1.734723475976814737E-16 ) ) ;
#22874=CARTESIAN_POINT ( 'NONE',  ( 31.81606138205700418, -21.15876147765404625, 76.30501292736998664 ) ) ;
#22882=CARTESIAN_POINT ( 'NONE',  ( 44.81606138205700063, -21.15876147765404625, 76.30501292736998664 ) ) ;
#22894=CARTESIAN_POINT ( 'NONE',  ( 30.81606138205700418, 40.39281886181299797, 80.75501292736983316 ) ) ;
#22896=CARTESIAN_POINT ( 'NONE',  ( 31.81606138205700418, -26.97987052895604876, 80.55501292737007191 ) ) ;
#22905=ORIENTED_EDGE ( 'NONE', *, *, #24961, .T. ) ;
#22908=CARTESIAN_POINT ( 'NONE',  ( 44.06606138205700063, 42.82479937715250173, 82.59790614618330551 ) ) ;
#22911=VERTEX_POINT ( 'NONE', #12601 ) ;
#22916=LINE ( 'NONE', #1143, #25447 ) ;
#22917=VECTOR ( 'NONE', #21281, 1000.000000000000114 ) ;
#22918=VECTOR ( 'NONE', #14074, 1000.000000000000000 ) ;
#22920=DIRECTION ( 'NONE',  ( -1.000000000000000000, 0.000000000000000000, 0.000000000000000000 ) ) ;
#22929=ORIENTED_EDGE ( 'NONE', *, *, #19961, .F. ) ;
#22934=VECTOR ( 'NONE', #3183, 1000.000000000000114 ) ;
#22944=ORIENTED_EDGE ( 'NONE', *, *, #15712, .T. ) ;
#22954=LINE ( 'NONE', #13308, #25271 ) ;
#22961=ADVANCED_FACE ( 'NONE', ( #9117, #5232, #9364 ), #11551, .T. ) ;
#22973=FACE_OUTER_BOUND ( 'NONE', #4960, .T. ) ;
#22977=ORIENTED_EDGE ( 'NONE', *, *, #2467, .T. ) ;
#22995=DIRECTION ( 'NONE',  ( 1.000000000000000000, 0.000000000000000000, 0.000000000000000000 ) ) ;
#23000=ORIENTED_EDGE ( 'NONE', *, *, #17938, .F. ) ;
#23002=CARTESIAN_POINT ( 'NONE',  ( 44.06606138205700063, 41.63025572888945192, 83.79244979444629848 ) ) ;
#23006=VECTOR ( 'NONE', #3062, 1000.000000000000000 ) ;
#23007=CARTESIAN_POINT ( 'NONE',  ( 38.44255644662678861, -39.60718113818700203, 84.30501292737011454 ) ) ;
#23015=LINE ( 'NONE', #13247, #16117 ) ;
#23024=ADVANCED_FACE ( 'NONE', ( #23247 ), #7552, .T. ) ;
#23025=DIRECTION ( 'NONE',  ( 0.000000000000000000, -1.000000000000000000, 0.000000000000000000 ) ) ;
#23029=CARTESIAN_POINT ( 'NONE',  ( 41.14099152588523367, -10.60718113818700026, 93.30501292736998664 ) ) ;
#23033=VECTOR ( 'NONE', #17942, 1000.000000000000000 ) ;
#23045=CARTESIAN_POINT ( 'NONE',  ( 40.64099152588522657, -1.357181138186998925, 79.30501292737000085 ) ) ;
#23056=ORIENTED_EDGE ( 'NONE', *, *, #3773, .T. ) ;
#23066=AXIS2_PLACEMENT_3D ( 'NONE', #3809, #2256, #19786 ) ;
#23068=PLANE ( 'NONE',  #600 ) ;
#23071=VECTOR ( 'NONE', #4731, 1000.000000000000114 ) ;
#23075=CARTESIAN_POINT ( 'NONE',  ( 40.64099152588522657, -1.357181138186998925, 80.05501292737000085 ) ) ;
#23077=ORIENTED_EDGE ( 'NONE', *, *, #20096, .T. ) ;
#23081=DIRECTION ( 'NONE',  ( 0.000000000000000000, -1.000000000000000000, 3.491481338843135327E-15 ) ) ;
#23087=CIRCLE ( 'NONE', #20212, 1.500000000000001332 ) ;
#23108=CIRCLE ( 'NONE', #16944, 1.500000000000001332 ) ;
#23117=CARTESIAN_POINT ( 'NONE',  ( 33.03722820848892638, 1.142818861812999742, 82.55501292736998664 ) ) ;
#23126=VECTOR ( 'NONE', #23667, 1000.000000000000000 ) ;
#23161=LINE ( 'NONE', #5650, #8880 ) ;
#23168=EDGE_CURVE ( 'NONE', #19007, #5938, #19771, .T. ) ;
#23175=VECTOR ( 'NONE', #21379, 1000.000000000000000 ) ;
#23190=CARTESIAN_POINT ( 'NONE',  ( 31.81606138205700418, 40.39281886181299797, 81.75501292736983316 ) ) ;
#23197=AXIS2_PLACEMENT_3D ( 'NONE', #14734, #20669, #17068 ) ;
#23198=CARTESIAN_POINT ( 'NONE',  ( 44.06606138205700063, -26.74044063519535186, 82.55501292737007191 ) ) ;
#23208=DIRECTION ( 'NONE',  ( -1.734723475976804876E-16, -3.491481338843135327E-15, -1.000000000000000000 ) ) ;
#23217=ORIENTED_EDGE ( 'NONE', *, *, #13806, .F. ) ;
#23222=CARTESIAN_POINT ( 'NONE',  ( 31.81606138205700418, 39.39281886181299797, 81.75501292736984738 ) ) ;
#23233=ADVANCED_FACE ( 'NONE', ( #14104 ), #4322, .F. ) ;
#23239=CYLINDRICAL_SURFACE ( 'NONE', #10446, 3.000000000000002665 ) ;
#23243=DIRECTION ( 'NONE',  ( 0.000000000000000000, -1.000000000000000000, 3.491481338843135327E-15 ) ) ;
#23247=FACE_OUTER_BOUND ( 'NONE', #18922, .T. ) ;
#23250=ORIENTED_EDGE ( 'NONE', *, *, #5796, .T. ) ;
#23251=LINE ( 'NONE', #15275, #17744 ) ;
#23254=AXIS2_PLACEMENT_3D ( 'NONE', #7336, #11466, #9783 ) ;
#23286=DIRECTION ( 'NONE',  ( 0.000000000000000000, -1.000000000000000000, 3.491481338843135327E-15 ) ) ;
#23299=ORIENTED_EDGE ( 'NONE', *, *, #8155, .T. ) ;
#23300=CARTESIAN_POINT ( 'NONE',  ( 30.81606138205700418, -31.45856502260510013, 77.07494475056050476 ) ) ;
#23303=ORIENTED_EDGE ( 'NONE', *, *, #17984, .F. ) ;
#23314=AXIS2_PLACEMENT_3D ( 'NONE', #2103, #17845, #173 ) ;
#23321=CYLINDRICAL_SURFACE ( 'NONE', #16437, 1.500000000000001332 ) ;
#23326=VERTEX_POINT ( 'NONE', #10623 ) ;
#23336=EDGE_CURVE ( 'NONE', #7351, #643, #18474, .T. ) ;
#23338=LINE ( 'NONE', #19229, #14283 ) ;
#23339=EDGE_CURVE ( 'NONE', #2531, #24390, #11229, .T. ) ;
#23361=DIRECTION ( 'NONE',  ( -1.734723475976804876E-16, -3.491481338843135327E-15, -1.000000000000000000 ) ) ;
#23368=CARTESIAN_POINT ( 'NONE',  ( 38.44255644662678861, -39.60718113818700203, 83.30501292737011454 ) ) ;
#23392=DIRECTION ( 'NONE',  ( 1.000000000000000000, 0.000000000000000000, 0.000000000000000000 ) ) ;
#23394=DIRECTION ( 'NONE',  ( 0.000000000000000000, -1.000000000000000000, 0.000000000000000000 ) ) ;
#23398=FACE_OUTER_BOUND ( 'NONE', #18995, .T. ) ;
#23418=LINE ( 'NONE', #13397, #2978 ) ;
#23428=LINE ( 'NONE', #11734, #7517 ) ;
#23450=EDGE_LOOP ( 'NONE', ( #15048, #6249, #25275, #1329, #21312, #2556, #10585, #10177, #19711, #18910, #24265, #17831, #24294, #11828, #11984, #16890 ) ) ;
#23473=VERTEX_POINT ( 'NONE', #934 ) ;
#23491=CARTESIAN_POINT ( 'NONE',  ( 32.56606138205700773, 41.63025572888945192, 83.79244979444629848 ) ) ;
#23502=EDGE_CURVE ( 'NONE', #1147, #23852, #21771, .T. ) ;
#23503=CARTESIAN_POINT ( 'NONE',  ( 35.64099152588523367, -8.167181138186998979, 88.30501292736998664 ) ) ;
#23528=CARTESIAN_POINT ( 'NONE',  ( 40.64099152588522657, 40.83281886181300280, 79.30501292736983032 ) ) ;
#23565=EDGE_CURVE ( 'NONE', #15554, #17064, #9898, .T. ) ;
#23584=CARTESIAN_POINT ( 'NONE',  ( 44.06606138205700063, 40.39281886181299797, 82.55501292736983032 ) ) ;
#23600=CIRCLE ( 'NONE', #9231, 4.000000000000003553 ) ;
#23613=VECTOR ( 'NONE', #6962, 1000.000000000000000 ) ;
#23621=CARTESIAN_POINT ( 'NONE',  ( 31.81606138205700418, -34.55876147765410167, 66.30501292737000085 ) ) ;
#23630=DIRECTION ( 'NONE',  ( 1.000000000000000000, -6.018531076210110289E-31, -1.734723475976804876E-16 ) ) ;
#23639=FACE_OUTER_BOUND ( 'NONE', #1596, .T. ) ;
#23644=LINE ( 'NONE', #5875, #24156 ) ;
#23651=EDGE_LOOP ( 'NONE', ( #204, #7853 ) ) ;
#23667=DIRECTION ( 'NONE',  ( -1.734723475976804876E-16, -3.552713678800500140E-15, -1.000000000000000000 ) ) ;
#23676=ORIENTED_EDGE ( 'NONE', *, *, #12903, .F. ) ;
#23685=CARTESIAN_POINT ( 'NONE',  ( 44.81606138205700063, -34.55876147765410167, 70.30501292737000085 ) ) ;
#23715=CARTESIAN_POINT ( 'NONE',  ( 32.56606138205700773, 40.39281886181299797, 82.55501292736983032 ) ) ;
#23718=AXIS2_PLACEMENT_3D ( 'NONE', #20174, #12079, #6639 ) ;
#23741=EDGE_CURVE ( 'NONE', #14213, #16039, #21897, .T. ) ;
#23751=FACE_OUTER_BOUND ( 'NONE', #21141, .T. ) ;
#23758=VERTEX_POINT ( 'NONE', #22271 ) ;
#23762=CIRCLE ( 'NONE', #9803, 10.00000000000000178 ) ;
#23765=VECTOR ( 'NONE', #6234, 1000.000000000000000 ) ;
#23782=DIRECTION ( 'NONE',  ( -1.510383499235849534E-16, -0.1218693434051499741, -0.9925461516413217611 ) ) ;
#23790=DIRECTION ( 'NONE',  ( 0.000000000000000000, -1.000000000000000000, 3.491481338843135327E-15 ) ) ;
#23815=CARTESIAN_POINT ( 'NONE',  ( 30.81606138205700418, -39.60718113818700203, 84.30501292737011454 ) ) ;
#23823=VECTOR ( 'NONE', #22077, 1000.000000000000000 ) ;
#23852=VERTEX_POINT ( 'NONE', #22143 ) ;
#23861=CARTESIAN_POINT ( 'NONE',  ( 38.31606138205699352, 43.35512946304240245, 81.37823623207320622 ) ) ;
#23865=EDGE_CURVE ( 'NONE', #2245, #4112, #8117, .T. ) ;
#23874=CIRCLE ( 'NONE', #12794, 4.000000000000000000 ) ;
#23876=CIRCLE ( 'NONE', #16073, 3.000000000000002665 ) ;
#23908=EDGE_CURVE ( 'NONE', #17348, #22306, #15047, .T. ) ;
#23916=ORIENTED_EDGE ( 'NONE', *, *, #8810, .F. ) ;
#23947=VECTOR ( 'NONE', #2291, 1000.000000000000000 ) ;
#23960=CIRCLE ( 'NONE', #17822, 1.750000000000001554 ) ;
#23970=VECTOR ( 'NONE', #5188, 1000.000000000000000 ) ;
#23983=LINE ( 'NONE', #14583, #17908 ) ;
#23997=DIRECTION ( 'NONE',  ( 0.000000000000000000, 1.000000000000000000, -6.938893903907402716E-15 ) ) ;
#24004=( GEOMETRIC_REPRESENTATION_CONTEXT ( 3 ) GLOBAL_UNCERTAINTY_ASSIGNED_CONTEXT ( ( #2499 ) ) GLOBAL_UNIT_ASSIGNED_CONTEXT ( ( #2755, #6638, #20306 ) ) REPRESENTATION_CONTEXT ( 'NONE', 'WORKASPACE' ) );
#24007=ORIENTED_EDGE ( 'NONE', *, *, #20361, .F. ) ;
#24015=ORIENTED_EDGE ( 'NONE', *, *, #20096, .F. ) ;
#24022=DIRECTION ( 'NONE',  ( 1.000000000000000000, 1.246695722929252133E-30, -1.734723475976824844E-16 ) ) ;
#24028=VECTOR ( 'NONE', #12842, 1000.000000000000000 ) ;
#24037=LINE ( 'NONE', #18136, #11092 ) ;
#24047=ADVANCED_FACE ( 'NONE', ( #16993 ), #24826, .T. ) ;
#24059=EDGE_CURVE ( 'NONE', #5938, #10765, #17244, .T. ) ;
#24061=DIRECTION ( 'NONE',  ( -5.047295537021760406E-31, 1.000000000000000000, -3.491481338843135327E-15 ) ) ;
#24079=DIRECTION ( 'NONE',  ( 0.000000000000000000, -1.000000000000000000, 3.491481338843135327E-15 ) ) ;
#24087=EDGE_CURVE ( 'NONE', #2531, #7462, #11716, .T. ) ;
#24105=DIRECTION ( 'NONE',  ( 0.000000000000000000, 1.000000000000000000, 0.000000000000000000 ) ) ;
#24133=ORIENTED_EDGE ( 'NONE', *, *, #491, .F. ) ;
#24145=ORIENTED_EDGE ( 'NONE', *, *, #6414, .F. ) ;
#24146=ORIENTED_EDGE ( 'NONE', *, *, #5779, .F. ) ;
#24156=VECTOR ( 'NONE', #15657, 1000.000000000000000 ) ;
#24157=DIRECTION ( 'NONE',  ( -1.000000000000000000, -1.734723475976804876E-16, 1.734723475976814737E-16 ) ) ;
#24170=VECTOR ( 'NONE', #14804, 1000.000000000000114 ) ;
#24173=LINE ( 'NONE', #12496, #10809 ) ;
#24190=VECTOR ( 'NONE', #2018, 1000.000000000000000 ) ;
#24207=DIRECTION ( 'NONE',  ( -1.933202721249430383E-16, 0.9925461516413217611, -0.1218693434051499741 ) ) ;
#24213=VERTEX_POINT ( 'NONE', #3834 ) ;
#24227=CARTESIAN_POINT ( 'NONE',  ( 45.81606138205700063, -34.55876147765410167, 70.30501292737000085 ) ) ;
#24228=CARTESIAN_POINT ( 'NONE',  ( 45.81606138205700063, -36.05876147765410877, 70.30501292737000085 ) ) ;
#24238=FACE_OUTER_BOUND ( 'NONE', #18792, .T. ) ;
#24243=DIRECTION ( 'NONE',  ( 1.000000000000000000, 1.734723475976804876E-16, -1.734723475976814737E-16 ) ) ;
#24263=CARTESIAN_POINT ( 'NONE',  ( 38.31606138205699352, 42.82479937715250173, 82.59790614618330551 ) ) ;
#24265=ORIENTED_EDGE ( 'NONE', *, *, #1627, .F. ) ;
#24268=ADVANCED_FACE ( 'NONE', ( #6287 ), #16438, .T. ) ;
#24271=FILL_AREA_STYLE ('',( #10644 ) ) ;
#24277=CARTESIAN_POINT ( 'NONE',  ( 17.31606138205699708, 34.87886987267149408, 78.19668729537065133 ) ) ;
#24289=ORIENTED_EDGE ( 'NONE', *, *, #5667, .F. ) ;
#24294=ORIENTED_EDGE ( 'NONE', *, *, #8448, .F. ) ;
#24295=ORIENTED_EDGE ( 'NONE', *, *, #2321, .F. ) ;
#24304=FACE_OUTER_BOUND ( 'NONE', #9914, .T. ) ;
#24308=DIRECTION ( 'NONE',  ( 0.000000000000000000, 1.000000000000000000, -4.625929269271481378E-15 ) ) ;
#24318=CARTESIAN_POINT ( 'NONE',  ( 38.41621794735363693, -36.60729675983900222, 83.30501292737011454 ) ) ;
#24319=EDGE_CURVE ( 'NONE', #2496, #20938, #17893, .T. ) ;
#24320=ORIENTED_EDGE ( 'NONE', *, *, #3014, .T. ) ;
#24324=ORIENTED_EDGE ( 'NONE', *, *, #1598, .T. ) ;
#24331=AXIS2_PLACEMENT_3D ( 'NONE', #10539, #22246, #12221 ) ;
#24339=ORIENTED_EDGE ( 'NONE', *, *, #2777, .F. ) ;
#24345=ORIENTED_EDGE ( 'NONE', *, *, #1650, .T. ) ;
#24352=ADVANCED_FACE ( 'NONE', ( #13888 ), #15937, .F. ) ;
#24356=CARTESIAN_POINT ( 'NONE',  ( 30.81606138205700418, 40.39281886181299797, 84.30501292736984453 ) ) ;
#24365=CIRCLE ( 'NONE', #20267, 2.000000000000001776 ) ;
#24366=ORIENTED_EDGE ( 'NONE', *, *, #8668, .F. ) ;
#24369=VECTOR ( 'NONE', #11911, 1000.000000000000000 ) ;
#24387=DIRECTION ( 'NONE',  ( -1.000000000000000000, 0.000000000000000000, 0.000000000000000000 ) ) ;
#24390=VERTEX_POINT ( 'NONE', #11037 ) ;
#24398=DIRECTION ( 'NONE',  ( -1.000000000000000000, 4.930380657631319405E-32, 1.734723475976804876E-16 ) ) ;
#24421=PLANE ( 'NONE',  #19301 ) ;
#24434=PLANE ( 'NONE',  #6892 ) ;
#24439=AXIS2_PLACEMENT_3D ( 'NONE', #3775, #11530, #9844 ) ;
#24440=CARTESIAN_POINT ( 'NONE',  ( 41.14099152588522657, -10.60718113818700026, 83.30501292737001506 ) ) ;
#24441=ORIENTED_EDGE ( 'NONE', *, *, #1948, .F. ) ;
#24452=FACE_OUTER_BOUND ( 'NONE', #21820, .T. ) ;
#24453=EDGE_CURVE ( 'NONE', #24213, #21678, #13106, .T. ) ;
#24466=ORIENTED_EDGE ( 'NONE', *, *, #8306, .F. ) ;
#24479=EDGE_CURVE ( 'NONE', #22728, #7783, #8730, .T. ) ;
#24493=ADVANCED_FACE ( 'NONE', ( #12845 ), #8862, .F. ) ;
#24496=DIRECTION ( 'NONE',  ( 1.000000000000000000, 1.734723475976805122E-16, -1.734723475976811039E-16 ) ) ;
#24500=DIRECTION ( 'NONE',  ( 1.734723475976814737E-16, -1.000000000000000000, 3.491481338843135327E-15 ) ) ;
#24509=VERTEX_POINT ( 'NONE', #14889 ) ;
#24512=DIRECTION ( 'NONE',  ( -1.734723475976814737E-16, 1.000000000000000000, -3.491481338843135327E-15 ) ) ;
#24528=CARTESIAN_POINT ( 'NONE',  ( 31.81606138205700418, 40.39281886181299797, 81.44836866983821722 ) ) ;
#24536=CARTESIAN_POINT ( 'NONE',  ( 45.81606138205700063, 40.39281886181299797, 81.44836866983821722 ) ) ;
#24545=FACE_OUTER_BOUND ( 'NONE', #1038, .T. ) ;
#24548=DIRECTION ( 'NONE',  ( 1.000000000000000000, 0.000000000000000000, -2.478176394252580155E-16 ) ) ;
#24551=DIRECTION ( 'NONE',  ( 1.734723475976814737E-16, -1.000000000000000000, 3.491481338843135327E-15 ) ) ;
#24557=VERTEX_POINT ( 'NONE', #23002 ) ;
#24565=CIRCLE ( 'NONE', #8138, 1.500000000000001332 ) ;
#24568=AXIS2_PLACEMENT_3D ( 'NONE', #11579, #3321, #9271 ) ;
#24572=FACE_OUTER_BOUND ( 'NONE', #5665, .T. ) ;
#24575=EDGE_CURVE ( 'NONE', #14052, #24723, #13731, .T. ) ;
#24590=EDGE_CURVE ( 'NONE', #11508, #9294, #23876, .T. ) ;
#24614=CARTESIAN_POINT ( 'NONE',  ( 31.81606138205700418, -31.45856502260510013, 77.07494475056050476 ) ) ;
#24628=EDGE_LOOP ( 'NONE', ( #5996, #19950, #20450, #16533 ) ) ;
#24632=AXIS2_PLACEMENT_3D ( 'NONE', #4219, #2140, #2396 ) ;
#24650=EDGE_CURVE ( 'NONE', #3225, #10140, #23251, .T. ) ;
#24667=CIRCLE ( 'NONE', #11950, 1.750000000000001554 ) ;
#24669=ORIENTED_EDGE ( 'NONE', *, *, #15060, .F. ) ;
#24672=DIRECTION ( 'NONE',  ( 1.000000000000000000, 1.734723475976804876E-16, -1.734723475976814737E-16 ) ) ;
#24691=ADVANCED_FACE ( 'NONE', ( #25038 ), #3545, .F. ) ;
#24692=CARTESIAN_POINT ( 'NONE',  ( 32.56606138205700773, 45.04446929126255128, 81.37823623207320622 ) ) ;
#24695=DIRECTION ( 'NONE',  ( -1.000000000000000000, -1.734723475976804876E-16, 1.734723475976814737E-16 ) ) ;
#24705=ORIENTED_EDGE ( 'NONE', *, *, #16991, .F. ) ;
#24707=PLANE ( 'NONE',  #25231 ) ;
#24723=VERTEX_POINT ( 'NONE', #15147 ) ;
#24729=ORIENTED_EDGE ( 'NONE', *, *, #23865, .F. ) ;
#24734=LINE ( 'NONE', #4922, #21712 ) ;
#24746=ORIENTED_EDGE ( 'NONE', *, *, #24479, .T. ) ;
#24747=DIRECTION ( 'NONE',  ( 1.000000000000000000, 2.168404344971005170E-16, -1.734723475976814737E-16 ) ) ;
#24753=FACE_OUTER_BOUND ( 'NONE', #21462, .T. ) ;
#24777=EDGE_LOOP ( 'NONE', ( #17047, #17318, #13270, #11123 ) ) ;
#24811=AXIS2_PLACEMENT_3D ( 'NONE', #23715, #6210, #6082 ) ;
#24813=ORIENTED_EDGE ( 'NONE', *, *, #4604, .F. ) ;
#24814=FACE_OUTER_BOUND ( 'NONE', #7519, .T. ) ;
#24826=CYLINDRICAL_SURFACE ( 'NONE', #16887, 1.750000000000001554 ) ;
#24828=EDGE_LOOP ( 'NONE', ( #3651, #22688, #4224, #11237 ) ) ;
#24890=VERTEX_POINT ( 'NONE', #9508 ) ;
#24908=DIRECTION ( 'NONE',  ( 0.000000000000000000, -1.000000000000000000, 3.491481338843135327E-15 ) ) ;
#24911=AXIS2_PLACEMENT_3D ( 'NONE', #18558, #17011, #14682 ) ;
#24921=VERTEX_POINT ( 'NONE', #19156 ) ;
#24922=DIRECTION ( 'NONE',  ( -1.734723475976804876E-16, -3.491481338843135327E-15, -1.000000000000000000 ) ) ;
#24946=FACE_OUTER_BOUND ( 'NONE', #5846, .T. ) ;
#24951=DIRECTION ( 'NONE',  ( -6.505213034913019208E-17, 1.000000000000000000, 0.000000000000000000 ) ) ;
#24961=EDGE_CURVE ( 'NONE', #19200, #4506, #17761, .T. ) ;
#24986=ORIENTED_EDGE ( 'NONE', *, *, #18532, .T. ) ;
#24992=CARTESIAN_POINT ( 'NONE',  ( 44.81606138205700063, -3.831401139557048197, 80.75501292737000369 ) ) ;
#25000=CARTESIAN_POINT ( 'NONE',  ( 30.81606138205700418, 40.39281886181299797, 66.30501292737000085 ) ) ;
#25011=DIRECTION ( 'NONE',  ( -1.000000000000000000, 0.000000000000000000, 0.000000000000000000 ) ) ;
#25038=FACE_OUTER_BOUND ( 'NONE', #2973, .T. ) ;
#25056=ORIENTED_EDGE ( 'NONE', *, *, #18853, .T. ) ;
#25059=DIRECTION ( 'NONE',  ( -1.000000000000000000, -1.734723475976814737E-16, 0.000000000000000000 ) ) ;
#25061=AXIS2_PLACEMENT_3D ( 'NONE', #1917, #13913, #3601 ) ;
#25076=( NAMED_UNIT ( * ) PLANE_ANGLE_UNIT ( ) SI_UNIT ( $, .RADIAN. ) );
#25083=DIRECTION ( 'NONE',  ( 0.000000000000000000, -1.000000000000000000, 3.469446951953701358E-15 ) ) ;
#25093=ORIENTED_EDGE ( 'NONE', *, *, #6282, .F. ) ;
#25106=EDGE_CURVE ( 'NONE', #21711, #643, #13997, .T. ) ;
#25136=CARTESIAN_POINT ( 'NONE',  ( 30.81606138205700418, -1.357181138186998925, 78.30501292736998664 ) ) ;
#25139=EDGE_CURVE ( 'NONE', #18087, #22306, #10133, .T. ) ;
#25141=EDGE_LOOP ( 'NONE', ( #24813, #13716, #18417, #1370 ) ) ;
#25143=PLANE ( 'NONE',  #24439 ) ;
#25144=PLANE ( 'NONE',  #21107 ) ;
#25153=CARTESIAN_POINT ( 'NONE',  ( 35.14099152588523367, -10.60718113818700026, 93.30501292736998664 ) ) ;
#25154=DIRECTION ( 'NONE',  ( 0.000000000000000000, -3.491481338843135327E-15, -1.000000000000000000 ) ) ;
#25159=DIRECTION ( 'NONE',  ( 0.000000000000000000, 1.000000000000000000, 0.000000000000000000 ) ) ;
#25171=EDGE_CURVE ( 'NONE', #22094, #14027, #23087, .T. ) ;
#25188=AXIS2_PLACEMENT_3D ( 'NONE', #4184, #22074, #17717 ) ;
#25197=ORIENTED_EDGE ( 'NONE', *, *, #24319, .F. ) ;
#25205=ADVANCED_FACE ( 'NONE', ( #2750 ), #18871, .T. ) ;
#25206=DIRECTION ( 'NONE',  ( 1.000000000000000000, 1.734723475976805122E-16, 0.000000000000000000 ) ) ;
#25209=( NAMED_UNIT ( * ) PLANE_ANGLE_UNIT ( ) SI_UNIT ( $, .RADIAN. ) );
#25211=DIRECTION ( 'NONE',  ( -1.000000000000000000, -1.734723475976799945E-16, 1.734723475976814737E-16 ) ) ;
#25219=AXIS2_PLACEMENT_3D ( 'NONE', #4046, #23630, #13841 ) ;
#25223=CARTESIAN_POINT ( 'NONE',  ( 44.81606138205700063, -21.15876147765410309, 66.30501292737000085 ) ) ;
#25231=AXIS2_PLACEMENT_3D ( 'NONE', #1140, #12769, #14935 ) ;
#25248=CARTESIAN_POINT ( 'NONE',  ( 45.81606138205700063, 34.87886987267150118, 81.44836866983821722 ) ) ;
#25252=VECTOR ( 'NONE', #3917, 1000.000000000000114 ) ;
#25253=DIRECTION ( 'NONE',  ( 0.000000000000000000, 1.000000000000000000, 0.000000000000000000 ) ) ;
#25267=ORIENTED_EDGE ( 'NONE', *, *, #11687, .F. ) ;
#25271=VECTOR ( 'NONE', #3501, 1000.000000000000000 ) ;
#25275=ORIENTED_EDGE ( 'NONE', *, *, #721, .F. ) ;
#25287=CARTESIAN_POINT ( 'NONE',  ( 44.81606138205700063, -34.67340937580780036, 71.26505871168839690 ) ) ;
#25303=VERTEX_POINT ( 'NONE', #15380 ) ;
#25310=ORIENTED_EDGE ( 'NONE', *, *, #13189, .F. ) ;
#25329=EDGE_LOOP ( 'NONE', ( #6011, #23303, #14360, #8569 ) ) ;
#25339=FACE_OUTER_BOUND ( 'NONE', #5496, .T. ) ;
#25347=CYLINDRICAL_SURFACE ( 'NONE', #11693, 3.999999999999996447 ) ;
#25368=AXIS2_PLACEMENT_3D ( 'NONE', #17856, #5998, #13852 ) ;
#25398=VERTEX_POINT ( 'NONE', #23621 ) ;
#25401=ORIENTED_EDGE ( 'NONE', *, *, #15385, .F. ) ;
#25406=LINE ( 'NONE', #5981, #25252 ) ;
#25411=FACE_OUTER_BOUND ( 'NONE', #11390, .T. ) ;
#25425=ORIENTED_EDGE ( 'NONE', *, *, #20592, .F. ) ;
#25434=ORIENTED_EDGE ( 'NONE', *, *, #18706, .T. ) ;
#25438=DIRECTION ( 'NONE',  ( -1.000000000000000000, -2.168404344971005170E-16, 1.734723475976814737E-16 ) ) ;
#25447=VECTOR ( 'NONE', #5025, 1000.000000000000000 ) ;
#25448=ORIENTED_EDGE ( 'NONE', *, *, #2982, .T. ) ;
#25455=VECTOR ( 'NONE', #5140, 1000.000000000000000 ) ;
#25481=CIRCLE ( 'NONE', #9494, 1.500000000000001332 ) ;
#25482=CARTESIAN_POINT ( 'NONE',  ( 31.81606138205700418, -30.95005513552129983, 81.04249030099066431 ) ) ;
ENDSEC;
END-ISO-10303-21;
